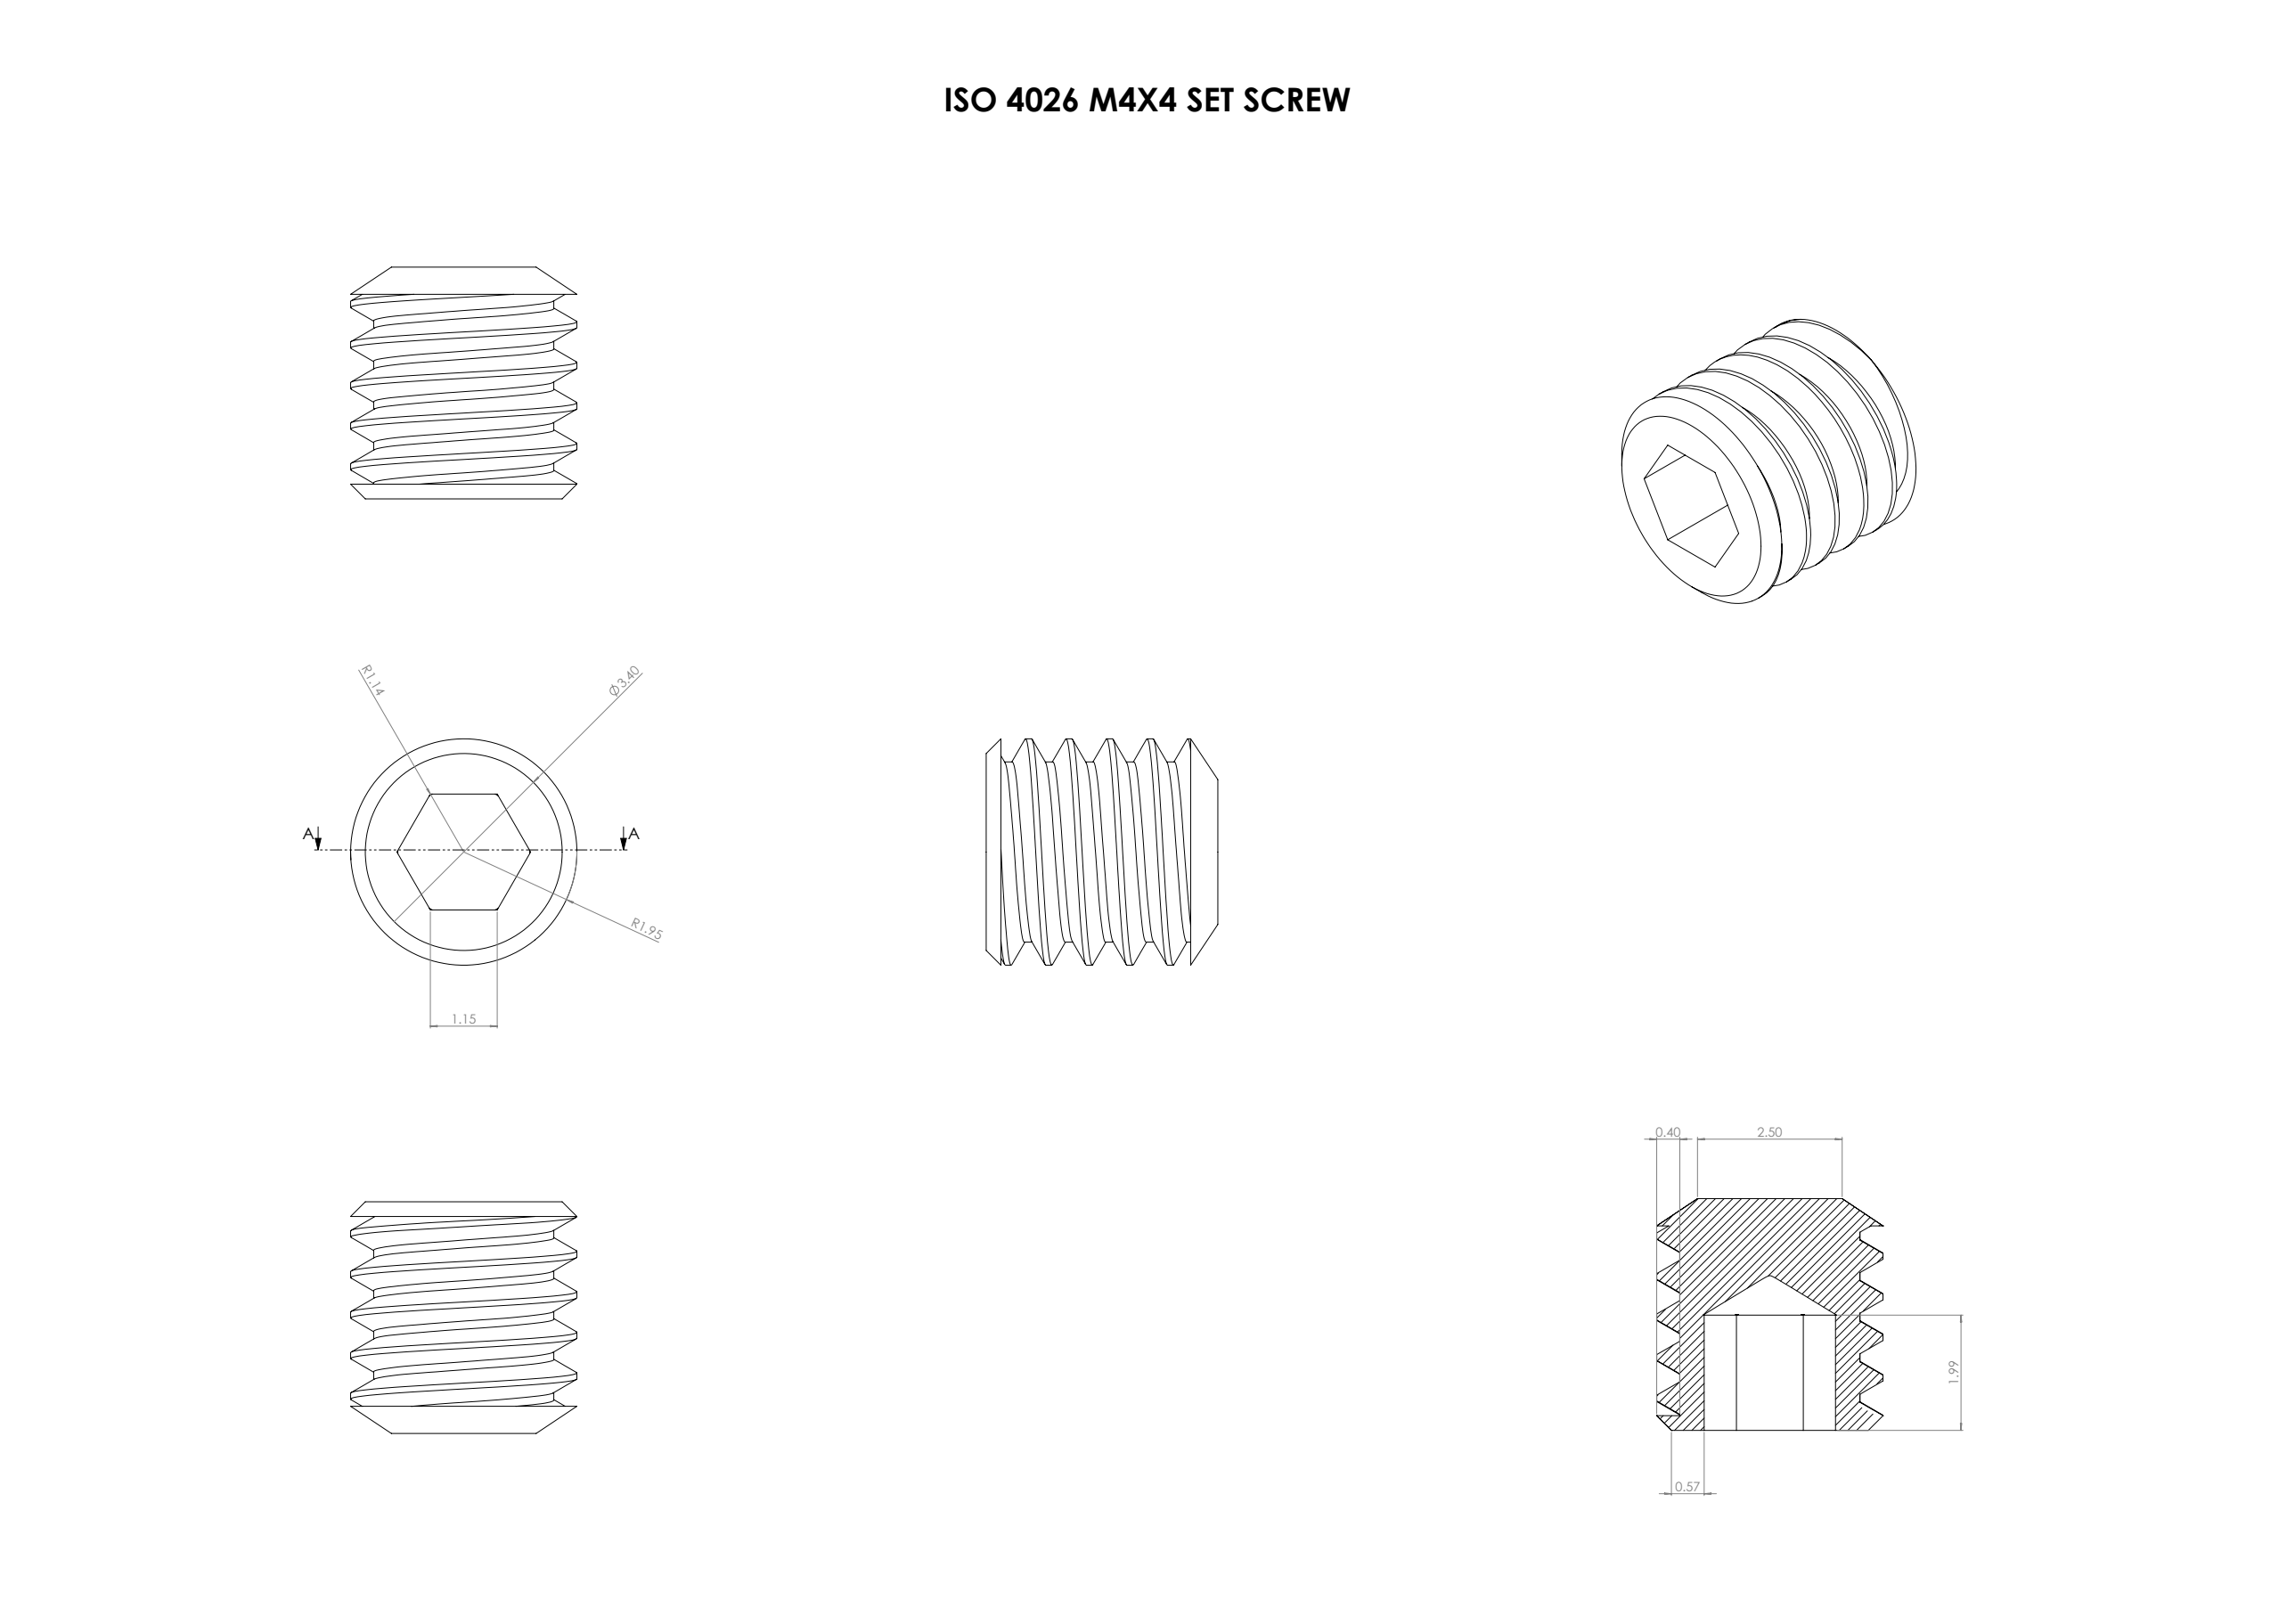
ISO-10303-21;
HEADER;
/* Generated by software containing ST-Developer
 * from STEP Tools, Inc. (www.steptools.com) 
 */

FILE_DESCRIPTION(
/* description */ (''),
/* implementation_level */ '2;1');

FILE_NAME(
/* name */ 
'14_ISO_4026_M4x4_Set_Screw.step',
/* time_stamp */ '2026-10-20T10:06:23-07:00',
/* author */ (''),
/* organization */ (''),
/* preprocessor_version */ 'ST-DEVELOPER v20.2',
/* originating_system */ 'Autodesk Translation Framework v15.15.0.0',
/* authorisation */ '');

FILE_SCHEMA (('AUTOMOTIVE_DESIGN { 1 0 10303 214 3 1 1 }'));
ENDSEC;

DATA;
#10=MECHANICAL_DESIGN_GEOMETRIC_PRESENTATION_REPRESENTATION('',(#467),#38611);
#118=(
BOUNDED_CURVE()
B_SPLINE_CURVE(2,(#26703,#26704,#26705),.UNSPECIFIED.,.F.,.F.)
B_SPLINE_CURVE_WITH_KNOTS((3,3),(0.,0.00350597452849922),.UNSPECIFIED.)
CURVE()
GEOMETRIC_REPRESENTATION_ITEM()
RATIONAL_B_SPLINE_CURVE((1.,1.00010739978215,1.))
REPRESENTATION_ITEM('')
);
#119=(
BOUNDED_CURVE()
B_SPLINE_CURVE(2,(#26707,#26708,#26709),.UNSPECIFIED.,.F.,.F.)
B_SPLINE_CURVE_WITH_KNOTS((3,3),(0.,0.00350597452849927),.UNSPECIFIED.)
CURVE()
GEOMETRIC_REPRESENTATION_ITEM()
RATIONAL_B_SPLINE_CURVE((1.,1.00010739978482,1.))
REPRESENTATION_ITEM('')
);
#120=(
BOUNDED_CURVE()
B_SPLINE_CURVE(2,(#26712,#26713,#26714),.UNSPECIFIED.,.F.,.F.)
B_SPLINE_CURVE_WITH_KNOTS((3,3),(0.,0.0035059745284993),.UNSPECIFIED.)
CURVE()
GEOMETRIC_REPRESENTATION_ITEM()
RATIONAL_B_SPLINE_CURVE((1.,1.00010739978303,1.))
REPRESENTATION_ITEM('')
);
#121=(
BOUNDED_CURVE()
B_SPLINE_CURVE(2,(#26716,#26717,#26718),.UNSPECIFIED.,.F.,.F.)
B_SPLINE_CURVE_WITH_KNOTS((3,3),(0.,0.00350597452849931),.UNSPECIFIED.)
CURVE()
GEOMETRIC_REPRESENTATION_ITEM()
RATIONAL_B_SPLINE_CURVE((1.,1.00010739978394,1.))
REPRESENTATION_ITEM('')
);
#122=(
BOUNDED_CURVE()
B_SPLINE_CURVE(2,(#26721,#26722,#26723),.UNSPECIFIED.,.F.,.F.)
B_SPLINE_CURVE_WITH_KNOTS((3,3),(0.,0.0035059745284993),.UNSPECIFIED.)
CURVE()
GEOMETRIC_REPRESENTATION_ITEM()
RATIONAL_B_SPLINE_CURVE((1.,1.00010739978631,1.))
REPRESENTATION_ITEM('')
);
#123=(
BOUNDED_CURVE()
B_SPLINE_CURVE(2,(#26725,#26726,#26727),.UNSPECIFIED.,.F.,.F.)
B_SPLINE_CURVE_WITH_KNOTS((3,3),(0.,0.00350597452849929),.UNSPECIFIED.)
CURVE()
GEOMETRIC_REPRESENTATION_ITEM()
RATIONAL_B_SPLINE_CURVE((1.,1.00010739978645,1.))
REPRESENTATION_ITEM('')
);
#124=(
BOUNDED_CURVE()
B_SPLINE_CURVE(2,(#26730,#26731,#26732),.UNSPECIFIED.,.F.,.F.)
B_SPLINE_CURVE_WITH_KNOTS((3,3),(0.,0.0035059745284993),.UNSPECIFIED.)
CURVE()
GEOMETRIC_REPRESENTATION_ITEM()
RATIONAL_B_SPLINE_CURVE((1.,1.00010739979569,1.))
REPRESENTATION_ITEM('')
);
#125=(
BOUNDED_CURVE()
B_SPLINE_CURVE(2,(#26734,#26735,#26736),.UNSPECIFIED.,.F.,.F.)
B_SPLINE_CURVE_WITH_KNOTS((3,3),(0.,0.0035059745284993),.UNSPECIFIED.)
CURVE()
GEOMETRIC_REPRESENTATION_ITEM()
RATIONAL_B_SPLINE_CURVE((1.,1.00010739979698,1.))
REPRESENTATION_ITEM('')
);
#126=(
BOUNDED_CURVE()
B_SPLINE_CURVE(2,(#26739,#26740,#26741),.UNSPECIFIED.,.F.,.F.)
B_SPLINE_CURVE_WITH_KNOTS((3,3),(0.,0.00350597452849928),.UNSPECIFIED.)
CURVE()
GEOMETRIC_REPRESENTATION_ITEM()
RATIONAL_B_SPLINE_CURVE((1.,1.00010739978256,1.))
REPRESENTATION_ITEM('')
);
#127=(
BOUNDED_CURVE()
B_SPLINE_CURVE(2,(#26743,#26744,#26745),.UNSPECIFIED.,.F.,.F.)
B_SPLINE_CURVE_WITH_KNOTS((3,3),(0.,0.00350597452849928),.UNSPECIFIED.)
CURVE()
GEOMETRIC_REPRESENTATION_ITEM()
RATIONAL_B_SPLINE_CURVE((1.,1.00010739978752,1.))
REPRESENTATION_ITEM('')
);
#128=(
BOUNDED_CURVE()
B_SPLINE_CURVE(2,(#26748,#26749,#26750),.UNSPECIFIED.,.F.,.F.)
B_SPLINE_CURVE_WITH_KNOTS((3,3),(0.,0.0035059745284993),.UNSPECIFIED.)
CURVE()
GEOMETRIC_REPRESENTATION_ITEM()
RATIONAL_B_SPLINE_CURVE((1.,1.0001073997843,1.))
REPRESENTATION_ITEM('')
);
#129=(
BOUNDED_CURVE()
B_SPLINE_CURVE(2,(#26752,#26753,#26754),.UNSPECIFIED.,.F.,.F.)
B_SPLINE_CURVE_WITH_KNOTS((3,3),(0.,0.00350597452849929),.UNSPECIFIED.)
CURVE()
GEOMETRIC_REPRESENTATION_ITEM()
RATIONAL_B_SPLINE_CURVE((1.,1.00010739978875,1.))
REPRESENTATION_ITEM('')
);
#439=SHAPE_REPRESENTATION_RELATIONSHIP('SRR','None',#38675,#453);
#453=ADVANCED_BREP_SHAPE_REPRESENTATION('',(#481),#38604);
#467=STYLED_ITEM('',(#38885),#481);
#481=MANIFOLD_SOLID_BREP('Set screw',#16241);
#499=B_SPLINE_SURFACE_WITH_KNOTS('',3,3,((#26238,#26239,#26240,#26241,#26242,
#26243,#26244,#26245,#26246,#26247,#26248,#26249,#26250,#26251,#26252,#26253,
#26254,#26255,#26256,#26257,#26258,#26259,#26260,#26261,#26262,#26263,#26264,
#26265,#26266,#26267,#26268,#26269,#26270,#26271,#26272),(#26273,#26274,
#26275,#26276,#26277,#26278,#26279,#26280,#26281,#26282,#26283,#26284,#26285,
#26286,#26287,#26288,#26289,#26290,#26291,#26292,#26293,#26294,#26295,#26296,
#26297,#26298,#26299,#26300,#26301,#26302,#26303,#26304,#26305,#26306,#26307),
(#26308,#26309,#26310,#26311,#26312,#26313,#26314,#26315,#26316,#26317,
#26318,#26319,#26320,#26321,#26322,#26323,#26324,#26325,#26326,#26327,#26328,
#26329,#26330,#26331,#26332,#26333,#26334,#26335,#26336,#26337,#26338,#26339,
#26340,#26341,#26342),(#26343,#26344,#26345,#26346,#26347,#26348,#26349,
#26350,#26351,#26352,#26353,#26354,#26355,#26356,#26357,#26358,#26359,#26360,
#26361,#26362,#26363,#26364,#26365,#26366,#26367,#26368,#26369,#26370,#26371,
#26372,#26373,#26374,#26375,#26376,#26377)),.UNSPECIFIED.,.F.,.F.,.F.,(4,
4),(4,1,1,1,1,1,1,1,1,1,1,1,1,1,1,1,1,1,1,1,1,1,1,1,1,1,1,1,1,1,1,1,4),
(0.,0.0460148164544132),(8.31058692273978,9.29422540264245,10.2778638825451,
11.2615023624478,12.2451408423505,13.2287793222531,14.2124178021558,15.1960562820585,
16.1796947619611,17.1633332418638,18.1469717217665,19.1306102016691,20.1142486815718,
21.0978871614745,22.0815256413772,23.0651641212798,24.0488026011825,25.0324410810852,
26.0160795609878,26.9997180408905,27.9833565207932,28.9669950006958,29.9506334805985,
30.9342719605012,31.9179104404039,32.9015489203065,33.8851874002092,34.8688258801119,
35.8524643600145,36.8361028399172,37.8197413198199,38.8033797997225,39.7870182796252),
 .UNSPECIFIED.);
#500=B_SPLINE_SURFACE_WITH_KNOTS('',3,3,((#26523,#26524,#26525,#26526,#26527,
#26528,#26529,#26530,#26531,#26532,#26533,#26534,#26535,#26536,#26537,#26538,
#26539,#26540,#26541,#26542,#26543,#26544,#26545,#26546,#26547,#26548,#26549,
#26550,#26551,#26552,#26553,#26554,#26555,#26556,#26557),(#26558,#26559,
#26560,#26561,#26562,#26563,#26564,#26565,#26566,#26567,#26568,#26569,#26570,
#26571,#26572,#26573,#26574,#26575,#26576,#26577,#26578,#26579,#26580,#26581,
#26582,#26583,#26584,#26585,#26586,#26587,#26588,#26589,#26590,#26591,#26592),
(#26593,#26594,#26595,#26596,#26597,#26598,#26599,#26600,#26601,#26602,
#26603,#26604,#26605,#26606,#26607,#26608,#26609,#26610,#26611,#26612,#26613,
#26614,#26615,#26616,#26617,#26618,#26619,#26620,#26621,#26622,#26623,#26624,
#26625,#26626,#26627),(#26628,#26629,#26630,#26631,#26632,#26633,#26634,
#26635,#26636,#26637,#26638,#26639,#26640,#26641,#26642,#26643,#26644,#26645,
#26646,#26647,#26648,#26649,#26650,#26651,#26652,#26653,#26654,#26655,#26656,
#26657,#26658,#26659,#26660,#26661,#26662)),.UNSPECIFIED.,.F.,.F.,.F.,(4,
4),(4,1,1,1,1,1,1,1,1,1,1,1,1,1,1,1,1,1,1,1,1,1,1,1,1,1,1,1,1,1,1,1,4),
(0.,0.0460148164544132),(11.6154215191106,12.5990599990133,13.582698478916,
14.5663369588187,15.5499754387213,16.533613918624,17.5172523985267,18.5008908784293,
19.484529358332,20.4681678382347,21.4518063181373,22.43544479804,23.4190832779427,
24.4027217578453,25.386360237748,26.3699987176507,27.3536371975534,28.337275677456,
29.3209141573587,30.3045526372614,31.288191117164,32.2718295970667,33.2554680769694,
34.239106556872,35.2227450367747,36.2063835166774,37.19002199658,38.1736604764827,
39.1572989563854,40.1409374362881,41.1245759161907,42.1082143960934,43.0918528759961),
 .UNSPECIFIED.);
#592=B_SPLINE_CURVE_WITH_KNOTS('',3,(#25799,#25800,#25801,#25802,#25803,
#25804,#25805,#25806,#25807,#25808),.UNSPECIFIED.,.F.,.F.,(4,3,3,4),(-4.09254174883832,
-3.93455391961068,-2.95091543970801,-2.06514013327811),.UNSPECIFIED.);
#593=B_SPLINE_CURVE_WITH_KNOTS('',3,(#25811,#25812,#25813,#25814,#25815,
#25816,#25817),.UNSPECIFIED.,.F.,.F.,(4,3,4),(0.,0.983638479902673,1.11419103802959),
 .UNSPECIFIED.);
#594=B_SPLINE_CURVE_WITH_KNOTS('',3,(#25822,#25823,#25824,#25825,#25826,
#25827,#25828,#25829,#25830,#25831,#25832,#25833,#25834,#25835,#25836,#25837,
#25838,#25839,#25840,#25841,#25842,#25843),.UNSPECIFIED.,.F.,.F.,(4,3,3,
3,3,3,3,4),(-10.3757270560179,-9.83638479902669,-8.85274631912402,-7.86910783922136,
-6.88546935931869,-5.90183087941602,-4.91819239951335,-4.09254174883832),
 .UNSPECIFIED.);
#595=B_SPLINE_CURVE_WITH_KNOTS('',3,(#25844,#25845,#25846,#25847,#25848,
#25849,#25850,#25851,#25852,#25853,#25854,#25855,#25856,#25857,#25858,#25859,
#25860,#25861,#25862,#25863,#25864,#25865),.UNSPECIFIED.,.F.,.F.,(4,3,3,
3,3,3,3,4),(1.11419103802959,1.96727695980534,2.95091543970801,3.93455391961068,
4.91819239951335,5.90183087941602,6.88546935931869,7.39737634520918),
 .UNSPECIFIED.);
#596=B_SPLINE_CURVE_WITH_KNOTS('',3,(#25870,#25871,#25872,#25873,#25874,
#25875,#25876,#25877,#25878,#25879,#25880,#25881,#25882,#25883,#25884,#25885,
#25886,#25887,#25888,#25889,#25890,#25891),.UNSPECIFIED.,.F.,.F.,(4,3,3,
3,3,3,3,4),(-16.6589123631975,-15.7382156784427,-14.75457719854,-13.7709387186374,
-12.7873002387347,-11.803661758832,-10.8200232789294,-10.3757270560179),
 .UNSPECIFIED.);
#597=B_SPLINE_CURVE_WITH_KNOTS('',3,(#25892,#25893,#25894,#25895,#25896,
#25897,#25898,#25899,#25900,#25901,#25902,#25903,#25904,#25905,#25906,#25907,
#25908,#25909,#25910,#25911,#25912,#25913),.UNSPECIFIED.,.F.,.F.,(4,3,3,
3,3,3,3,4),(7.39737634520918,7.86910783922136,8.85274631912403,9.83638479902669,
10.8200232789294,11.803661758832,12.7873002387347,13.6805616523888),
 .UNSPECIFIED.);
#598=B_SPLINE_CURVE_WITH_KNOTS('',3,(#25918,#25919,#25920,#25921,#25922,
#25923,#25924,#25925,#25926,#25927,#25928,#25929,#25930,#25931,#25932,#25933,
#25934,#25935,#25936,#25937,#25938,#25939,#25940,#25941,#25942),
 .UNSPECIFIED.,.F.,.F.,(4,3,3,3,3,3,3,3,4),(-22.9420976703771,-22.6236850377614,
-21.6400465578587,-20.6564080779561,-19.6727695980534,-18.6891311181507,
-17.705492638248,-16.7218541583454,-16.6589123631975),.UNSPECIFIED.);
#599=B_SPLINE_CURVE_WITH_KNOTS('',3,(#25943,#25944,#25945,#25946,#25947,
#25948,#25949,#25950,#25951,#25952,#25953,#25954,#25955,#25956,#25957,#25958,
#25959,#25960,#25961,#25962,#25963,#25964,#25965,#25966,#25967),
 .UNSPECIFIED.,.F.,.F.,(4,3,3,3,3,3,3,3,4),(13.6805616523888,13.7709387186374,
14.75457719854,15.7382156784427,16.7218541583454,17.705492638248,18.6891311181507,
19.6727695980534,19.9637469595684),.UNSPECIFIED.);
#600=B_SPLINE_CURVE_WITH_KNOTS('',3,(#25972,#25973,#25974,#25975,#25976,
#25977,#25978,#25979,#25980,#25981,#25982,#25983,#25984,#25985,#25986,#25987,
#25988,#25989,#25990,#25991,#25992,#25993),.UNSPECIFIED.,.F.,.F.,(4,3,3,
3,3,3,3,4),(-29.2252829775567,-28.5255159171774,-27.5418774372747,-26.5582389573721,
-25.5746004774694,-24.5909619975667,-23.6073235176641,-22.9420976703771),
 .UNSPECIFIED.);
#601=B_SPLINE_CURVE_WITH_KNOTS('',3,(#25994,#25995,#25996,#25997,#25998,
#25999,#26000,#26001,#26002,#26003,#26004,#26005,#26006,#26007,#26008,#26009,
#26010,#26011,#26012,#26013,#26014,#26015),.UNSPECIFIED.,.F.,.F.,(4,3,3,
3,3,3,3,4),(19.9637469595684,20.6564080779561,21.6400465578587,22.6236850377614,
23.6073235176641,24.5909619975667,25.5746004774694,26.2469322667479),
 .UNSPECIFIED.);
#602=B_SPLINE_CURVE_WITH_KNOTS('',3,(#26021,#26022,#26023,#26024),
 .UNSPECIFIED.,.F.,.F.,(4,4),(40.8407044966673,41.026712742718),
 .UNSPECIFIED.);
#603=B_SPLINE_CURVE_WITH_KNOTS('',3,(#26030,#26031,#26032,#26033,#26034,
#26035,#26036,#26037,#26038,#26039),.UNSPECIFIED.,.F.,.F.,(4,1,1,1,1,1,
1,4),(34.5575191894877,35.2227450367747,36.2063835166774,37.19002199658,
38.1736604764827,39.1572989563854,40.1409374362881,40.8407044966673),
 .UNSPECIFIED.);
#604=B_SPLINE_CURVE_WITH_KNOTS('',3,(#26042,#26043,#26044,#26045,#26046,
#26047,#26048,#26049,#26050),.UNSPECIFIED.,.F.,.F.,(4,1,1,1,1,1,4),(34.5575191894877,
34.8688258801119,35.8524643600145,36.8361028399172,37.8197413198199,38.8033797997225,
39.7870182796252),.UNSPECIFIED.);
#605=B_SPLINE_CURVE_WITH_KNOTS('',3,(#26055,#26056,#26057,#26058,#26059,
#26060,#26061,#26062,#26063,#26064,#26065),.UNSPECIFIED.,.F.,.F.,(4,1,1,
1,1,1,1,1,4),(28.2743338823081,28.337275677456,29.3209141573587,30.3045526372614,
31.288191117164,32.2718295970667,33.2554680769694,34.239106556872,34.5575191894877),
 .UNSPECIFIED.);
#606=B_SPLINE_CURVE_WITH_KNOTS('',3,(#26066,#26067,#26068,#26069,#26070,
#26071,#26072,#26073,#26074,#26075),.UNSPECIFIED.,.F.,.F.,(4,1,1,1,1,1,
1,4),(28.2743338823081,28.9669950006958,29.9506334805985,30.9342719605012,
31.9179104404039,32.9015489203065,33.8851874002092,34.5575191894877),
 .UNSPECIFIED.);
#607=B_SPLINE_CURVE_WITH_KNOTS('',3,(#26080,#26081,#26082,#26083,#26084,
#26085,#26086,#26087,#26088,#26089),.UNSPECIFIED.,.F.,.F.,(4,1,1,1,1,1,
1,4),(21.9911485751285,22.43544479804,23.4190832779427,24.4027217578453,
25.386360237748,26.3699987176507,27.3536371975534,28.2743338823081),
 .UNSPECIFIED.);
#608=B_SPLINE_CURVE_WITH_KNOTS('',3,(#26090,#26091,#26092,#26093,#26094,
#26095,#26096,#26097,#26098,#26099,#26100),.UNSPECIFIED.,.F.,.F.,(4,1,1,
1,1,1,1,1,4),(21.9911485751285,22.0815256413772,23.0651641212798,24.0488026011825,
25.0324410810852,26.0160795609878,26.9997180408905,27.9833565207932,28.2743338823081),
 .UNSPECIFIED.);
#609=B_SPLINE_CURVE_WITH_KNOTS('',3,(#26105,#26106,#26107,#26108,#26109,
#26110,#26111,#26112,#26113,#26114),.UNSPECIFIED.,.F.,.F.,(4,1,1,1,1,1,
1,4),(15.707963267949,16.533613918624,17.5172523985267,18.5008908784293,
19.484529358332,20.4681678382347,21.4518063181373,21.9911485751285),
 .UNSPECIFIED.);
#610=B_SPLINE_CURVE_WITH_KNOTS('',3,(#26115,#26116,#26117,#26118,#26119,
#26120,#26121,#26122,#26123,#26124),.UNSPECIFIED.,.F.,.F.,(4,1,1,1,1,1,
1,4),(15.707963267949,16.1796947619611,17.1633332418638,18.1469717217665,
19.1306102016691,20.1142486815718,21.0978871614745,21.9911485751285),
 .UNSPECIFIED.);
#611=B_SPLINE_CURVE_WITH_KNOTS('',3,(#26127,#26128,#26129,#26130,#26131,
#26132,#26133,#26134,#26135,#26136,#26137,#26138,#26139,#26140,#26141,#26142,
#26143,#26144,#26145,#26146,#26147,#26148,#26149,#26150,#26151,#26152,#26153,
#26154,#26155,#26156,#26157,#26158,#26159,#26160,#26161,#26162,#26163,#26164,
#26165,#26166,#26167,#26168,#26169,#26170,#26171,#26172,#26173,#26174,#26175,
#26176,#26177,#26178),.UNSPECIFIED.,.F.,.F.,(4,3,3,3,3,3,3,3,3,3,3,3,3,
3,3,3,3,4),(-0.366397579005848,-0.350883706971702,-0.330766239349036,-0.315517000142461,
-0.286726965402577,-0.272902702918689,-0.237792065049709,-0.221751325260965,
-0.207725190445974,-0.184643803987141,-0.160983363133761,-0.147813025816132,
-0.137069449159236,-0.102802086869427,-0.0797357051045986,-0.0678496931522027,
-0.0293463862030034,0.),.UNSPECIFIED.);
#612=B_SPLINE_CURVE_WITH_KNOTS('',3,(#26183,#26184,#26185,#26186,#26187,
#26188,#26189,#26190,#26191,#26192,#26193,#26194,#26195,#26196,#26197,#26198,
#26199,#26200,#26201,#26202,#26203,#26204,#26205,#26206,#26207,#26208,#26209,
#26210,#26211,#26212,#26213,#26214,#26215,#26216,#26217,#26218,#26219,#26220,
#26221,#26222,#26223,#26224,#26225,#26226,#26227,#26228,#26229,#26230,#26231,
#26232,#26233,#26234,#26235,#26236,#26237),.UNSPECIFIED.,.F.,.F.,(4,3,3,
3,3,3,3,3,3,3,3,3,3,3,3,3,3,3,4),(-0.364629307890673,-0.34556327172486,
-0.316373806239452,-0.304392727635835,-0.282581484008551,-0.264372375760159,
-0.252241992724549,-0.215817384559742,-0.198585804821849,-0.187223821335194,
-0.163761333129925,-0.14297227179632,-0.127520914102002,-0.116250236265464,
-0.0871876771990984,-0.0683674864494023,-0.0546742414735358,-0.0223329481946053,
0.),.UNSPECIFIED.);
#613=B_SPLINE_CURVE_WITH_KNOTS('',3,(#26378,#26379,#26380,#26381,#26382,
#26383,#26384,#26385,#26386,#26387,#26388,#26389,#26390),.UNSPECIFIED.,
 .F.,.F.,(4,3,3,3,4),(26.2469322667479,26.5582389573721,27.5418774372747,
28.5255159171774,29.4112912236073),.UNSPECIFIED.);
#614=B_SPLINE_CURVE_WITH_KNOTS('',3,(#26392,#26393,#26394,#26395,#26396,
#26397,#26398,#26399,#26400,#26401,#26402,#26403,#26404,#26405,#26406,#26407,
#26408,#26409,#26410,#26411,#26412,#26413,#26414,#26415,#26416,#26417,#26418,
#26419,#26420,#26421,#26422,#26423,#26424,#26425,#26426,#26427,#26428,#26429,
#26430,#26431,#26432,#26433,#26434,#26435,#26436,#26437,#26438,#26439,#26440,
#26441,#26442,#26443),.UNSPECIFIED.,.F.,.F.,(4,3,3,3,3,3,3,3,3,3,3,3,3,
3,3,3,3,4),(-0.366397579005841,-0.350883706971692,-0.330766244233555,-0.315517008906463,
-0.286727928129561,-0.272902925597775,-0.237792297289449,-0.221751641342226,
-0.207725209589122,-0.184643803987137,-0.160983359465905,-0.147812972159593,
-0.137069363910321,-0.102802022932741,-0.0797355322205692,-0.0678497129848781,
-0.0293463878428536,0.),.UNSPECIFIED.);
#615=B_SPLINE_CURVE_WITH_KNOTS('',3,(#26444,#26445,#26446,#26447,#26448,
#26449,#26450,#26451,#26452),.UNSPECIFIED.,.F.,.F.,(4,1,1,1,1,1,4),(10.3757270560179,
11.2615023624478,12.2451408423505,13.2287793222531,14.2124178021558,15.1960562820585,
15.707963267949),.UNSPECIFIED.);
#616=B_SPLINE_CURVE_WITH_KNOTS('',3,(#26458,#26459,#26460,#26461,#26462,
#26463,#26464,#26465,#26466,#26467,#26468,#26469,#26470,#26471,#26472,#26473,
#26474,#26475,#26476,#26477,#26478,#26479,#26480,#26481,#26482,#26483,#26484,
#26485,#26486,#26487,#26488,#26489,#26490,#26491,#26492,#26493,#26494,#26495,
#26496,#26497,#26498,#26499,#26500,#26501,#26502,#26503,#26504,#26505,#26506,
#26507,#26508,#26509,#26510,#26511,#26512),.UNSPECIFIED.,.F.,.F.,(4,3,3,
3,3,3,3,3,3,3,3,3,3,3,3,3,3,3,4),(-0.364629307890667,-0.345563271724857,
-0.316373785930453,-0.304392687069709,-0.282581361533379,-0.264370838693491,
-0.252241562212899,-0.215816938962755,-0.198585271532288,-0.18722386611403,
-0.163761333129928,-0.142972181196261,-0.127520768604021,-0.116250225520689,
-0.087187669140517,-0.0683674708033287,-0.0546742449026845,-0.0223330177554359,
0.),.UNSPECIFIED.);
#617=B_SPLINE_CURVE_WITH_KNOTS('',3,(#26515,#26516,#26517,#26518,#26519,
#26520,#26521,#26522),.UNSPECIFIED.,.F.,.F.,(4,1,1,1,1,4),(11.6154215191106,
12.5990599990133,13.582698478916,14.5663369588187,15.5499754387213,15.707963267949),
 .UNSPECIFIED.);
#618=B_SPLINE_CURVE_WITH_KNOTS('',3,(#26663,#26664,#26665,#26666,#26667,
#26668,#26669,#26670,#26671,#26672),.UNSPECIFIED.,.F.,.F.,(4,3,3,4),(-31.4764313568854,
-30.4927928769827,-29.5091543970801,-29.2252829775567),.UNSPECIFIED.);
#930=CYLINDRICAL_SURFACE('',#16910,0.1954);
#931=CYLINDRICAL_SURFACE('',#16912,0.1954);
#932=CYLINDRICAL_SURFACE('',#16913,0.1954);
#933=CYLINDRICAL_SURFACE('',#16914,0.1954);
#934=CYLINDRICAL_SURFACE('',#16915,0.1954);
#935=CYLINDRICAL_SURFACE('',#16916,0.15555);
#936=CYLINDRICAL_SURFACE('',#16918,0.15555);
#937=CYLINDRICAL_SURFACE('',#16920,0.15555);
#938=CYLINDRICAL_SURFACE('',#16921,0.15555);
#939=CYLINDRICAL_SURFACE('',#16922,0.15555);
#940=CYLINDRICAL_SURFACE('',#16930,0.15555);
#941=CYLINDRICAL_SURFACE('',#16978,0.1954);
#1187=FACE_BOUND('',#3096,.T.);
#1386=CIRCLE('',#16911,0.1954);
#1387=CIRCLE('',#16917,0.15555);
#1388=CIRCLE('',#16919,0.15555);
#1389=CIRCLE('',#16924,0.1954);
#1390=CIRCLE('',#16925,0.1954);
#1391=CIRCLE('',#16927,0.1954);
#1392=CIRCLE('',#16928,0.1954);
#1393=CIRCLE('',#16929,0.15555);
#1394=CIRCLE('',#16932,0.115470053837925);
#1395=CIRCLE('',#16934,0.115470053837925);
#1396=CIRCLE('',#16936,0.115470053837925);
#1397=CIRCLE('',#16938,0.115470053837925);
#1398=CIRCLE('',#16940,0.115470053837925);
#1399=CIRCLE('',#16942,0.115470053837925);
#1400=CIRCLE('',#16944,0.113827101150665);
#1401=CIRCLE('',#16945,0.113827101150665);
#1402=CIRCLE('',#16946,0.113827101150665);
#1403=CIRCLE('',#16947,0.113827101150665);
#1404=CIRCLE('',#16948,0.113827101150665);
#1405=CIRCLE('',#16949,0.113827101150665);
#1406=CIRCLE('',#16950,0.113827101150665);
#1407=CIRCLE('',#16976,0.125);
#1408=CIRCLE('',#16979,0.1954);
#1409=CIRCLE('',#16981,0.17);
#1743=CONICAL_SURFACE('',#16943,0.0577350269189626,1.02403331474479);
#1744=CONICAL_SURFACE('',#16977,0.1625,0.982793723247329);
#1745=CONICAL_SURFACE('',#16980,0.185,0.785398163397449);
#2100=FACE_OUTER_BOUND('',#3045,.T.);
#2101=FACE_OUTER_BOUND('',#3046,.T.);
#2102=FACE_OUTER_BOUND('',#3047,.T.);
#2103=FACE_OUTER_BOUND('',#3048,.T.);
#2104=FACE_OUTER_BOUND('',#3049,.T.);
#2105=FACE_OUTER_BOUND('',#3050,.T.);
#2106=FACE_OUTER_BOUND('',#3051,.T.);
#2107=FACE_OUTER_BOUND('',#3052,.T.);
#2108=FACE_OUTER_BOUND('',#3053,.T.);
#2109=FACE_OUTER_BOUND('',#3054,.T.);
#2110=FACE_OUTER_BOUND('',#3055,.T.);
#2111=FACE_OUTER_BOUND('',#3056,.T.);
#2112=FACE_OUTER_BOUND('',#3057,.T.);
#2113=FACE_OUTER_BOUND('',#3058,.T.);
#2114=FACE_OUTER_BOUND('',#3059,.T.);
#2115=FACE_OUTER_BOUND('',#3060,.T.);
#2116=FACE_OUTER_BOUND('',#3061,.T.);
#2117=FACE_OUTER_BOUND('',#3062,.T.);
#2118=FACE_OUTER_BOUND('',#3063,.T.);
#2119=FACE_OUTER_BOUND('',#3064,.T.);
#2120=FACE_OUTER_BOUND('',#3065,.T.);
#2121=FACE_OUTER_BOUND('',#3066,.T.);
#2122=FACE_OUTER_BOUND('',#3067,.T.);
#2123=FACE_OUTER_BOUND('',#3068,.T.);
#2124=FACE_OUTER_BOUND('',#3069,.T.);
#2125=FACE_OUTER_BOUND('',#3070,.T.);
#2126=FACE_OUTER_BOUND('',#3071,.T.);
#2127=FACE_OUTER_BOUND('',#3072,.T.);
#2128=FACE_OUTER_BOUND('',#3073,.T.);
#2129=FACE_OUTER_BOUND('',#3074,.T.);
#2130=FACE_OUTER_BOUND('',#3075,.T.);
#2131=FACE_OUTER_BOUND('',#3076,.T.);
#2132=FACE_OUTER_BOUND('',#3077,.T.);
#2133=FACE_OUTER_BOUND('',#3078,.T.);
#2134=FACE_OUTER_BOUND('',#3079,.T.);
#2135=FACE_OUTER_BOUND('',#3080,.T.);
#2136=FACE_OUTER_BOUND('',#3081,.T.);
#2137=FACE_OUTER_BOUND('',#3082,.T.);
#2138=FACE_OUTER_BOUND('',#3083,.T.);
#2139=FACE_OUTER_BOUND('',#3084,.T.);
#2140=FACE_OUTER_BOUND('',#3085,.T.);
#2141=FACE_OUTER_BOUND('',#3086,.T.);
#2142=FACE_OUTER_BOUND('',#3087,.T.);
#2143=FACE_OUTER_BOUND('',#3088,.T.);
#2144=FACE_OUTER_BOUND('',#3089,.T.);
#2145=FACE_OUTER_BOUND('',#3090,.T.);
#2146=FACE_OUTER_BOUND('',#3091,.T.);
#2147=FACE_OUTER_BOUND('',#3092,.T.);
#2148=FACE_OUTER_BOUND('',#3093,.T.);
#2149=FACE_OUTER_BOUND('',#3094,.T.);
#2150=FACE_OUTER_BOUND('',#3095,.T.);
#3045=EDGE_LOOP('',(#11601,#11602,#11603,#11604));
#3046=EDGE_LOOP('',(#11605,#11606,#11607,#11608));
#3047=EDGE_LOOP('',(#11609,#11610,#11611,#11612));
#3048=EDGE_LOOP('',(#11613,#11614,#11615,#11616));
#3049=EDGE_LOOP('',(#11617,#11618,#11619,#11620));
#3050=EDGE_LOOP('',(#11621,#11622,#11623));
#3051=EDGE_LOOP('',(#11624,#11625,#11626,#11627,#11628));
#3052=EDGE_LOOP('',(#11629,#11630,#11631,#11632));
#3053=EDGE_LOOP('',(#11633,#11634,#11635,#11636));
#3054=EDGE_LOOP('',(#11637,#11638,#11639,#11640));
#3055=EDGE_LOOP('',(#11641,#11642,#11643,#11644,#11645,#11646));
#3056=EDGE_LOOP('',(#11647,#11648,#11649,#11650,#11651,#11652,#11653,#11654,
#11655,#11656,#11657,#11658,#11659));
#3057=EDGE_LOOP('',(#11660,#11661,#11662,#11663,#11664));
#3058=EDGE_LOOP('',(#11665,#11666,#11667,#11668));
#3059=EDGE_LOOP('',(#11669,#11670,#11671,#11672,#11673,#11674,#11675,#11676,
#11677,#11678,#11679,#11680,#11681,#11682));
#3060=EDGE_LOOP('',(#11683,#11684));
#3061=EDGE_LOOP('',(#11685,#11686));
#3062=EDGE_LOOP('',(#11687,#11688));
#3063=EDGE_LOOP('',(#11689,#11690));
#3064=EDGE_LOOP('',(#11691,#11692));
#3065=EDGE_LOOP('',(#11693,#11694));
#3066=EDGE_LOOP('',(#11695,#11696,#11697,#11698,#11699,#11700,#11701,#11702,
#11703,#11704,#11705,#11706,#11707,#11708,#11709,#11710,#11711,#11712,#11713,
#11714,#11715,#11716,#11717,#11718,#11719,#11720,#11721));
#3067=EDGE_LOOP('',(#11722,#11723,#11724,#11725));
#3068=EDGE_LOOP('',(#11726,#11727,#11728));
#3069=EDGE_LOOP('',(#11729,#11730,#11731,#11732));
#3070=EDGE_LOOP('',(#11733,#11734,#11735));
#3071=EDGE_LOOP('',(#11736,#11737,#11738));
#3072=EDGE_LOOP('',(#11739,#11740,#11741,#11742));
#3073=EDGE_LOOP('',(#11743,#11744,#11745));
#3074=EDGE_LOOP('',(#11746,#11747,#11748,#11749));
#3075=EDGE_LOOP('',(#11750,#11751,#11752));
#3076=EDGE_LOOP('',(#11753,#11754,#11755));
#3077=EDGE_LOOP('',(#11756,#11757,#11758));
#3078=EDGE_LOOP('',(#11759,#11760,#11761));
#3079=EDGE_LOOP('',(#11762,#11763,#11764));
#3080=EDGE_LOOP('',(#11765,#11766,#11767));
#3081=EDGE_LOOP('',(#11768,#11769,#11770));
#3082=EDGE_LOOP('',(#11771,#11772,#11773,#11774));
#3083=EDGE_LOOP('',(#11775,#11776,#11777,#11778));
#3084=EDGE_LOOP('',(#11779,#11780,#11781));
#3085=EDGE_LOOP('',(#11782,#11783,#11784));
#3086=EDGE_LOOP('',(#11785,#11786,#11787));
#3087=EDGE_LOOP('',(#11788,#11789,#11790,#11791));
#3088=EDGE_LOOP('',(#11792,#11793,#11794));
#3089=EDGE_LOOP('',(#11795,#11796,#11797));
#3090=EDGE_LOOP('',(#11798,#11799,#11800));
#3091=EDGE_LOOP('',(#11801));
#3092=EDGE_LOOP('',(#11802,#11803,#11804,#11805,#11806,#11807));
#3093=EDGE_LOOP('',(#11808,#11809,#11810,#11811));
#3094=EDGE_LOOP('',(#11812,#11813,#11814,#11815,#11816,#11817));
#3095=EDGE_LOOP('',(#11818));
#3096=EDGE_LOOP('',(#11819,#11820,#11821,#11822,#11823,#11824));
#4162=LINE('',#25797,#5386);
#4163=LINE('',#25821,#5387);
#4164=LINE('',#25869,#5388);
#4165=LINE('',#25917,#5389);
#4166=LINE('',#25971,#5390);
#4167=LINE('',#26019,#5391);
#4168=LINE('',#26029,#5392);
#4169=LINE('',#26054,#5393);
#4170=LINE('',#26079,#5394);
#4171=LINE('',#26104,#5395);
#4172=LINE('',#26676,#5396);
#4173=LINE('',#26680,#5397);
#4174=LINE('',#26684,#5398);
#4175=LINE('',#26688,#5399);
#4176=LINE('',#26692,#5400);
#4177=LINE('',#26695,#5401);
#4178=LINE('',#26700,#5402);
#4179=LINE('',#26758,#5403);
#4180=LINE('',#26760,#5404);
#4181=LINE('',#26761,#5405);
#4182=LINE('',#26764,#5406);
#4183=LINE('',#26765,#5407);
#4184=LINE('',#26768,#5408);
#4185=LINE('',#26769,#5409);
#4186=LINE('',#26772,#5410);
#4187=LINE('',#26773,#5411);
#4188=LINE('',#26776,#5412);
#4189=LINE('',#26777,#5413);
#4190=LINE('',#26780,#5414);
#4191=LINE('',#26781,#5415);
#4192=LINE('',#26784,#5416);
#4193=LINE('',#26785,#5417);
#4194=LINE('',#26788,#5418);
#4195=LINE('',#26789,#5419);
#4196=LINE('',#26792,#5420);
#4197=LINE('',#26793,#5421);
#4198=LINE('',#26795,#5422);
#4199=LINE('',#26797,#5423);
#4200=LINE('',#26800,#5424);
#4201=LINE('',#26803,#5425);
#4202=LINE('',#26804,#5426);
#4203=LINE('',#26806,#5427);
#4204=LINE('',#26808,#5428);
#4205=LINE('',#26811,#5429);
#4206=LINE('',#26812,#5430);
#4207=LINE('',#26814,#5431);
#4208=LINE('',#26818,#5432);
#4209=LINE('',#26826,#5433);
#4210=LINE('',#26832,#5434);
#5386=VECTOR('',#19329,0.2);
#5387=VECTOR('',#19334,0.2);
#5388=VECTOR('',#19337,0.2);
#5389=VECTOR('',#19340,0.2);
#5390=VECTOR('',#19343,0.2);
#5391=VECTOR('',#19346,0.15555);
#5392=VECTOR('',#19351,0.15555);
#5393=VECTOR('',#19356,0.15555);
#5394=VECTOR('',#19359,0.15555);
#5395=VECTOR('',#19362,0.15555);
#5396=VECTOR('',#19381,1.);
#5397=VECTOR('',#19386,1.);
#5398=VECTOR('',#19391,1.);
#5399=VECTOR('',#19396,1.);
#5400=VECTOR('',#19401,1.);
#5401=VECTOR('',#19406,1.);
#5402=VECTOR('',#19411,0.0577350269189626);
#5403=VECTOR('',#19428,1.);
#5404=VECTOR('',#19429,1.);
#5405=VECTOR('',#19430,1.);
#5406=VECTOR('',#19433,1.);
#5407=VECTOR('',#19434,1.);
#5408=VECTOR('',#19437,1.);
#5409=VECTOR('',#19438,1.);
#5410=VECTOR('',#19441,1.);
#5411=VECTOR('',#19442,1.);
#5412=VECTOR('',#19445,1.);
#5413=VECTOR('',#19446,1.);
#5414=VECTOR('',#19449,1.);
#5415=VECTOR('',#19450,1.);
#5416=VECTOR('',#19453,1.);
#5417=VECTOR('',#19454,1.);
#5418=VECTOR('',#19457,1.);
#5419=VECTOR('',#19458,1.);
#5420=VECTOR('',#19461,1.);
#5421=VECTOR('',#19462,1.);
#5422=VECTOR('',#19465,1.);
#5423=VECTOR('',#19468,1.);
#5424=VECTOR('',#19473,1.);
#5425=VECTOR('',#19476,1.);
#5426=VECTOR('',#19477,1.);
#5427=VECTOR('',#19480,1.);
#5428=VECTOR('',#19483,1.);
#5429=VECTOR('',#19486,1.);
#5430=VECTOR('',#19487,1.);
#5431=VECTOR('',#19490,1.);
#5432=VECTOR('',#19497,1.);
#5433=VECTOR('',#19510,0.1625);
#5434=VECTOR('',#19519,0.185);
#6589=VERTEX_POINT('',#25795);
#6590=VERTEX_POINT('',#25796);
#6591=VERTEX_POINT('',#25798);
#6592=VERTEX_POINT('',#25809);
#6593=VERTEX_POINT('',#25819);
#6594=VERTEX_POINT('',#25820);
#6595=VERTEX_POINT('',#25867);
#6596=VERTEX_POINT('',#25868);
#6597=VERTEX_POINT('',#25915);
#6598=VERTEX_POINT('',#25916);
#6599=VERTEX_POINT('',#25969);
#6600=VERTEX_POINT('',#25970);
#6601=VERTEX_POINT('',#26017);
#6602=VERTEX_POINT('',#26018);
#6603=VERTEX_POINT('',#26020);
#6604=VERTEX_POINT('',#26027);
#6605=VERTEX_POINT('',#26028);
#6606=VERTEX_POINT('',#26040);
#6607=VERTEX_POINT('',#26052);
#6608=VERTEX_POINT('',#26053);
#6609=VERTEX_POINT('',#26077);
#6610=VERTEX_POINT('',#26078);
#6611=VERTEX_POINT('',#26102);
#6612=VERTEX_POINT('',#26103);
#6613=VERTEX_POINT('',#26126);
#6614=VERTEX_POINT('',#26179);
#6615=VERTEX_POINT('',#26181);
#6616=VERTEX_POINT('',#26391);
#6617=VERTEX_POINT('',#26454);
#6618=VERTEX_POINT('',#26457);
#6619=VERTEX_POINT('',#26674);
#6620=VERTEX_POINT('',#26675);
#6621=VERTEX_POINT('',#26679);
#6622=VERTEX_POINT('',#26683);
#6623=VERTEX_POINT('',#26687);
#6624=VERTEX_POINT('',#26691);
#6625=VERTEX_POINT('',#26698);
#6626=VERTEX_POINT('',#26699);
#6627=VERTEX_POINT('',#26701);
#6628=VERTEX_POINT('',#26706);
#6629=VERTEX_POINT('',#26710);
#6630=VERTEX_POINT('',#26715);
#6631=VERTEX_POINT('',#26719);
#6632=VERTEX_POINT('',#26724);
#6633=VERTEX_POINT('',#26728);
#6634=VERTEX_POINT('',#26733);
#6635=VERTEX_POINT('',#26737);
#6636=VERTEX_POINT('',#26742);
#6637=VERTEX_POINT('',#26746);
#6638=VERTEX_POINT('',#26751);
#6639=VERTEX_POINT('',#26757);
#6640=VERTEX_POINT('',#26759);
#6641=VERTEX_POINT('',#26763);
#6642=VERTEX_POINT('',#26767);
#6643=VERTEX_POINT('',#26771);
#6644=VERTEX_POINT('',#26775);
#6645=VERTEX_POINT('',#26779);
#6646=VERTEX_POINT('',#26783);
#6647=VERTEX_POINT('',#26787);
#6648=VERTEX_POINT('',#26791);
#6649=VERTEX_POINT('',#26802);
#6650=VERTEX_POINT('',#26810);
#6651=VERTEX_POINT('',#26823);
#6652=VERTEX_POINT('',#26830);
#8416=EDGE_CURVE('',#6589,#6590,#4162,.T.);
#8417=EDGE_CURVE('',#6589,#6591,#592,.T.);
#8418=EDGE_CURVE('',#6591,#6592,#1386,.T.);
#8419=EDGE_CURVE('',#6592,#6590,#593,.T.);
#8420=EDGE_CURVE('',#6593,#6594,#4163,.T.);
#8421=EDGE_CURVE('',#6593,#6589,#594,.T.);
#8422=EDGE_CURVE('',#6590,#6594,#595,.T.);
#8423=EDGE_CURVE('',#6595,#6596,#4164,.T.);
#8424=EDGE_CURVE('',#6595,#6593,#596,.T.);
#8425=EDGE_CURVE('',#6594,#6596,#597,.T.);
#8426=EDGE_CURVE('',#6597,#6598,#4165,.T.);
#8427=EDGE_CURVE('',#6597,#6595,#598,.T.);
#8428=EDGE_CURVE('',#6596,#6598,#599,.T.);
#8429=EDGE_CURVE('',#6599,#6600,#4166,.T.);
#8430=EDGE_CURVE('',#6599,#6597,#600,.T.);
#8431=EDGE_CURVE('',#6598,#6600,#601,.T.);
#8432=EDGE_CURVE('',#6601,#6602,#4167,.T.);
#8433=EDGE_CURVE('',#6601,#6603,#602,.T.);
#8434=EDGE_CURVE('',#6602,#6603,#1387,.T.);
#8435=EDGE_CURVE('',#6604,#6605,#4168,.T.);
#8436=EDGE_CURVE('',#6604,#6601,#603,.T.);
#8437=EDGE_CURVE('',#6606,#6602,#1388,.T.);
#8438=EDGE_CURVE('',#6605,#6606,#604,.T.);
#8439=EDGE_CURVE('',#6607,#6608,#4169,.T.);
#8440=EDGE_CURVE('',#6607,#6604,#605,.T.);
#8441=EDGE_CURVE('',#6608,#6605,#606,.T.);
#8442=EDGE_CURVE('',#6609,#6610,#4170,.T.);
#8443=EDGE_CURVE('',#6609,#6607,#607,.T.);
#8444=EDGE_CURVE('',#6610,#6608,#608,.T.);
#8445=EDGE_CURVE('',#6611,#6612,#4171,.T.);
#8446=EDGE_CURVE('',#6611,#6609,#609,.T.);
#8447=EDGE_CURVE('',#6612,#6610,#610,.T.);
#8448=EDGE_CURVE('',#6603,#6613,#611,.T.);
#8449=EDGE_CURVE('',#6614,#6613,#1389,.F.);
#8450=EDGE_CURVE('',#6615,#6614,#1390,.F.);
#8451=EDGE_CURVE('',#6615,#6606,#612,.T.);
#8452=EDGE_CURVE('',#6600,#6615,#613,.T.);
#8453=EDGE_CURVE('',#6616,#6592,#614,.T.);
#8454=EDGE_CURVE('',#6616,#6612,#615,.T.);
#8455=EDGE_CURVE('',#6592,#6617,#1391,.T.);
#8456=EDGE_CURVE('',#6617,#6591,#1392,.T.);
#8457=EDGE_CURVE('',#6591,#6618,#616,.T.);
#8458=EDGE_CURVE('',#6618,#6616,#1393,.T.);
#8459=EDGE_CURVE('',#6618,#6611,#617,.T.);
#8460=EDGE_CURVE('',#6613,#6599,#618,.T.);
#8461=EDGE_CURVE('',#6619,#6620,#4172,.T.);
#8462=EDGE_CURVE('',#6620,#6619,#1394,.T.);
#8463=EDGE_CURVE('',#6620,#6621,#4173,.T.);
#8464=EDGE_CURVE('',#6621,#6620,#1395,.T.);
#8465=EDGE_CURVE('',#6621,#6622,#4174,.T.);
#8466=EDGE_CURVE('',#6622,#6621,#1396,.T.);
#8467=EDGE_CURVE('',#6622,#6623,#4175,.T.);
#8468=EDGE_CURVE('',#6623,#6622,#1397,.T.);
#8469=EDGE_CURVE('',#6623,#6624,#4176,.T.);
#8470=EDGE_CURVE('',#6624,#6623,#1398,.T.);
#8471=EDGE_CURVE('',#6624,#6619,#4177,.T.);
#8472=EDGE_CURVE('',#6619,#6624,#1399,.T.);
#8473=EDGE_CURVE('',#6625,#6626,#4178,.T.);
#8474=EDGE_CURVE('',#6627,#6626,#1400,.T.);
#8475=EDGE_CURVE('',#6621,#6627,#118,.T.);
#8476=EDGE_CURVE('',#6628,#6620,#119,.T.);
#8477=EDGE_CURVE('',#6629,#6628,#1401,.T.);
#8478=EDGE_CURVE('',#6620,#6629,#120,.T.);
#8479=EDGE_CURVE('',#6630,#6619,#121,.T.);
#8480=EDGE_CURVE('',#6631,#6630,#1402,.T.);
#8481=EDGE_CURVE('',#6619,#6631,#122,.T.);
#8482=EDGE_CURVE('',#6632,#6624,#123,.T.);
#8483=EDGE_CURVE('',#6633,#6632,#1403,.T.);
#8484=EDGE_CURVE('',#6624,#6633,#124,.T.);
#8485=EDGE_CURVE('',#6634,#6623,#125,.T.);
#8486=EDGE_CURVE('',#6635,#6634,#1404,.T.);
#8487=EDGE_CURVE('',#6623,#6635,#126,.T.);
#8488=EDGE_CURVE('',#6636,#6622,#127,.T.);
#8489=EDGE_CURVE('',#6637,#6636,#1405,.T.);
#8490=EDGE_CURVE('',#6622,#6637,#128,.T.);
#8491=EDGE_CURVE('',#6638,#6621,#129,.T.);
#8492=EDGE_CURVE('',#6626,#6638,#1406,.T.);
#8493=EDGE_CURVE('',#6639,#6622,#4179,.T.);
#8494=EDGE_CURVE('',#6640,#6639,#4180,.T.);
#8495=EDGE_CURVE('',#6640,#6621,#4181,.T.);
#8496=EDGE_CURVE('',#6621,#6641,#4182,.T.);
#8497=EDGE_CURVE('',#6641,#6638,#4183,.T.);
#8498=EDGE_CURVE('',#6642,#6623,#4184,.T.);
#8499=EDGE_CURVE('',#6639,#6642,#4185,.T.);
#8500=EDGE_CURVE('',#6635,#6643,#4186,.T.);
#8501=EDGE_CURVE('',#6623,#6643,#4187,.T.);
#8502=EDGE_CURVE('',#6622,#6644,#4188,.T.);
#8503=EDGE_CURVE('',#6644,#6636,#4189,.T.);
#8504=EDGE_CURVE('',#6645,#6640,#4190,.T.);
#8505=EDGE_CURVE('',#6645,#6620,#4191,.T.);
#8506=EDGE_CURVE('',#6620,#6646,#4192,.T.);
#8507=EDGE_CURVE('',#6646,#6628,#4193,.T.);
#8508=EDGE_CURVE('',#6647,#6624,#4194,.T.);
#8509=EDGE_CURVE('',#6642,#6647,#4195,.T.);
#8510=EDGE_CURVE('',#6633,#6648,#4196,.T.);
#8511=EDGE_CURVE('',#6624,#6648,#4197,.T.);
#8512=EDGE_CURVE('',#6643,#6634,#4198,.T.);
#8513=EDGE_CURVE('',#6637,#6644,#4199,.T.);
#8514=EDGE_CURVE('',#6648,#6632,#4200,.T.);
#8515=EDGE_CURVE('',#6649,#6630,#4201,.T.);
#8516=EDGE_CURVE('',#6631,#6649,#4202,.T.);
#8517=EDGE_CURVE('',#6629,#6646,#4203,.T.);
#8518=EDGE_CURVE('',#6627,#6641,#4204,.T.);
#8519=EDGE_CURVE('',#6650,#6619,#4205,.T.);
#8520=EDGE_CURVE('',#6647,#6650,#4206,.T.);
#8521=EDGE_CURVE('',#6619,#6649,#4207,.T.);
#8522=EDGE_CURVE('',#6650,#6645,#4208,.T.);
#8523=EDGE_CURVE('',#6651,#6651,#1407,.T.);
#8524=EDGE_CURVE('',#6617,#6651,#4209,.T.);
#8525=EDGE_CURVE('',#6613,#6615,#1408,.F.);
#8526=EDGE_CURVE('',#6652,#6652,#1409,.T.);
#8527=EDGE_CURVE('',#6652,#6614,#4210,.T.);
#11601=ORIENTED_EDGE('',*,*,#8416,.F.);
#11602=ORIENTED_EDGE('',*,*,#8417,.T.);
#11603=ORIENTED_EDGE('',*,*,#8418,.T.);
#11604=ORIENTED_EDGE('',*,*,#8419,.T.);
#11605=ORIENTED_EDGE('',*,*,#8420,.F.);
#11606=ORIENTED_EDGE('',*,*,#8421,.T.);
#11607=ORIENTED_EDGE('',*,*,#8416,.T.);
#11608=ORIENTED_EDGE('',*,*,#8422,.T.);
#11609=ORIENTED_EDGE('',*,*,#8423,.F.);
#11610=ORIENTED_EDGE('',*,*,#8424,.T.);
#11611=ORIENTED_EDGE('',*,*,#8420,.T.);
#11612=ORIENTED_EDGE('',*,*,#8425,.T.);
#11613=ORIENTED_EDGE('',*,*,#8426,.F.);
#11614=ORIENTED_EDGE('',*,*,#8427,.T.);
#11615=ORIENTED_EDGE('',*,*,#8423,.T.);
#11616=ORIENTED_EDGE('',*,*,#8428,.T.);
#11617=ORIENTED_EDGE('',*,*,#8429,.F.);
#11618=ORIENTED_EDGE('',*,*,#8430,.T.);
#11619=ORIENTED_EDGE('',*,*,#8426,.T.);
#11620=ORIENTED_EDGE('',*,*,#8431,.T.);
#11621=ORIENTED_EDGE('',*,*,#8432,.F.);
#11622=ORIENTED_EDGE('',*,*,#8433,.T.);
#11623=ORIENTED_EDGE('',*,*,#8434,.F.);
#11624=ORIENTED_EDGE('',*,*,#8435,.F.);
#11625=ORIENTED_EDGE('',*,*,#8436,.T.);
#11626=ORIENTED_EDGE('',*,*,#8432,.T.);
#11627=ORIENTED_EDGE('',*,*,#8437,.F.);
#11628=ORIENTED_EDGE('',*,*,#8438,.F.);
#11629=ORIENTED_EDGE('',*,*,#8439,.F.);
#11630=ORIENTED_EDGE('',*,*,#8440,.T.);
#11631=ORIENTED_EDGE('',*,*,#8435,.T.);
#11632=ORIENTED_EDGE('',*,*,#8441,.F.);
#11633=ORIENTED_EDGE('',*,*,#8442,.F.);
#11634=ORIENTED_EDGE('',*,*,#8443,.T.);
#11635=ORIENTED_EDGE('',*,*,#8439,.T.);
#11636=ORIENTED_EDGE('',*,*,#8444,.F.);
#11637=ORIENTED_EDGE('',*,*,#8445,.F.);
#11638=ORIENTED_EDGE('',*,*,#8446,.T.);
#11639=ORIENTED_EDGE('',*,*,#8442,.T.);
#11640=ORIENTED_EDGE('',*,*,#8447,.F.);
#11641=ORIENTED_EDGE('',*,*,#8437,.T.);
#11642=ORIENTED_EDGE('',*,*,#8434,.T.);
#11643=ORIENTED_EDGE('',*,*,#8448,.T.);
#11644=ORIENTED_EDGE('',*,*,#8449,.F.);
#11645=ORIENTED_EDGE('',*,*,#8450,.F.);
#11646=ORIENTED_EDGE('',*,*,#8451,.T.);
#11647=ORIENTED_EDGE('',*,*,#8451,.F.);
#11648=ORIENTED_EDGE('',*,*,#8452,.F.);
#11649=ORIENTED_EDGE('',*,*,#8431,.F.);
#11650=ORIENTED_EDGE('',*,*,#8428,.F.);
#11651=ORIENTED_EDGE('',*,*,#8425,.F.);
#11652=ORIENTED_EDGE('',*,*,#8422,.F.);
#11653=ORIENTED_EDGE('',*,*,#8419,.F.);
#11654=ORIENTED_EDGE('',*,*,#8453,.F.);
#11655=ORIENTED_EDGE('',*,*,#8454,.T.);
#11656=ORIENTED_EDGE('',*,*,#8447,.T.);
#11657=ORIENTED_EDGE('',*,*,#8444,.T.);
#11658=ORIENTED_EDGE('',*,*,#8441,.T.);
#11659=ORIENTED_EDGE('',*,*,#8438,.T.);
#11660=ORIENTED_EDGE('',*,*,#8455,.T.);
#11661=ORIENTED_EDGE('',*,*,#8456,.T.);
#11662=ORIENTED_EDGE('',*,*,#8457,.T.);
#11663=ORIENTED_EDGE('',*,*,#8458,.T.);
#11664=ORIENTED_EDGE('',*,*,#8453,.T.);
#11665=ORIENTED_EDGE('',*,*,#8445,.T.);
#11666=ORIENTED_EDGE('',*,*,#8454,.F.);
#11667=ORIENTED_EDGE('',*,*,#8458,.F.);
#11668=ORIENTED_EDGE('',*,*,#8459,.T.);
#11669=ORIENTED_EDGE('',*,*,#8448,.F.);
#11670=ORIENTED_EDGE('',*,*,#8433,.F.);
#11671=ORIENTED_EDGE('',*,*,#8436,.F.);
#11672=ORIENTED_EDGE('',*,*,#8440,.F.);
#11673=ORIENTED_EDGE('',*,*,#8443,.F.);
#11674=ORIENTED_EDGE('',*,*,#8446,.F.);
#11675=ORIENTED_EDGE('',*,*,#8459,.F.);
#11676=ORIENTED_EDGE('',*,*,#8457,.F.);
#11677=ORIENTED_EDGE('',*,*,#8417,.F.);
#11678=ORIENTED_EDGE('',*,*,#8421,.F.);
#11679=ORIENTED_EDGE('',*,*,#8424,.F.);
#11680=ORIENTED_EDGE('',*,*,#8427,.F.);
#11681=ORIENTED_EDGE('',*,*,#8430,.F.);
#11682=ORIENTED_EDGE('',*,*,#8460,.F.);
#11683=ORIENTED_EDGE('',*,*,#8461,.F.);
#11684=ORIENTED_EDGE('',*,*,#8462,.F.);
#11685=ORIENTED_EDGE('',*,*,#8463,.F.);
#11686=ORIENTED_EDGE('',*,*,#8464,.F.);
#11687=ORIENTED_EDGE('',*,*,#8465,.F.);
#11688=ORIENTED_EDGE('',*,*,#8466,.F.);
#11689=ORIENTED_EDGE('',*,*,#8467,.F.);
#11690=ORIENTED_EDGE('',*,*,#8468,.F.);
#11691=ORIENTED_EDGE('',*,*,#8469,.F.);
#11692=ORIENTED_EDGE('',*,*,#8470,.F.);
#11693=ORIENTED_EDGE('',*,*,#8471,.F.);
#11694=ORIENTED_EDGE('',*,*,#8472,.F.);
#11695=ORIENTED_EDGE('',*,*,#8473,.T.);
#11696=ORIENTED_EDGE('',*,*,#8474,.F.);
#11697=ORIENTED_EDGE('',*,*,#8475,.F.);
#11698=ORIENTED_EDGE('',*,*,#8464,.T.);
#11699=ORIENTED_EDGE('',*,*,#8476,.F.);
#11700=ORIENTED_EDGE('',*,*,#8477,.F.);
#11701=ORIENTED_EDGE('',*,*,#8478,.F.);
#11702=ORIENTED_EDGE('',*,*,#8462,.T.);
#11703=ORIENTED_EDGE('',*,*,#8479,.F.);
#11704=ORIENTED_EDGE('',*,*,#8480,.F.);
#11705=ORIENTED_EDGE('',*,*,#8481,.F.);
#11706=ORIENTED_EDGE('',*,*,#8472,.T.);
#11707=ORIENTED_EDGE('',*,*,#8482,.F.);
#11708=ORIENTED_EDGE('',*,*,#8483,.F.);
#11709=ORIENTED_EDGE('',*,*,#8484,.F.);
#11710=ORIENTED_EDGE('',*,*,#8470,.T.);
#11711=ORIENTED_EDGE('',*,*,#8485,.F.);
#11712=ORIENTED_EDGE('',*,*,#8486,.F.);
#11713=ORIENTED_EDGE('',*,*,#8487,.F.);
#11714=ORIENTED_EDGE('',*,*,#8468,.T.);
#11715=ORIENTED_EDGE('',*,*,#8488,.F.);
#11716=ORIENTED_EDGE('',*,*,#8489,.F.);
#11717=ORIENTED_EDGE('',*,*,#8490,.F.);
#11718=ORIENTED_EDGE('',*,*,#8466,.T.);
#11719=ORIENTED_EDGE('',*,*,#8491,.F.);
#11720=ORIENTED_EDGE('',*,*,#8492,.F.);
#11721=ORIENTED_EDGE('',*,*,#8473,.F.);
#11722=ORIENTED_EDGE('',*,*,#8465,.T.);
#11723=ORIENTED_EDGE('',*,*,#8493,.F.);
#11724=ORIENTED_EDGE('',*,*,#8494,.F.);
#11725=ORIENTED_EDGE('',*,*,#8495,.T.);
#11726=ORIENTED_EDGE('',*,*,#8491,.T.);
#11727=ORIENTED_EDGE('',*,*,#8496,.T.);
#11728=ORIENTED_EDGE('',*,*,#8497,.T.);
#11729=ORIENTED_EDGE('',*,*,#8467,.T.);
#11730=ORIENTED_EDGE('',*,*,#8498,.F.);
#11731=ORIENTED_EDGE('',*,*,#8499,.F.);
#11732=ORIENTED_EDGE('',*,*,#8493,.T.);
#11733=ORIENTED_EDGE('',*,*,#8487,.T.);
#11734=ORIENTED_EDGE('',*,*,#8500,.T.);
#11735=ORIENTED_EDGE('',*,*,#8501,.F.);
#11736=ORIENTED_EDGE('',*,*,#8488,.T.);
#11737=ORIENTED_EDGE('',*,*,#8502,.T.);
#11738=ORIENTED_EDGE('',*,*,#8503,.T.);
#11739=ORIENTED_EDGE('',*,*,#8463,.T.);
#11740=ORIENTED_EDGE('',*,*,#8495,.F.);
#11741=ORIENTED_EDGE('',*,*,#8504,.F.);
#11742=ORIENTED_EDGE('',*,*,#8505,.T.);
#11743=ORIENTED_EDGE('',*,*,#8476,.T.);
#11744=ORIENTED_EDGE('',*,*,#8506,.T.);
#11745=ORIENTED_EDGE('',*,*,#8507,.T.);
#11746=ORIENTED_EDGE('',*,*,#8469,.T.);
#11747=ORIENTED_EDGE('',*,*,#8508,.F.);
#11748=ORIENTED_EDGE('',*,*,#8509,.F.);
#11749=ORIENTED_EDGE('',*,*,#8498,.T.);
#11750=ORIENTED_EDGE('',*,*,#8484,.T.);
#11751=ORIENTED_EDGE('',*,*,#8510,.T.);
#11752=ORIENTED_EDGE('',*,*,#8511,.F.);
#11753=ORIENTED_EDGE('',*,*,#8485,.T.);
#11754=ORIENTED_EDGE('',*,*,#8501,.T.);
#11755=ORIENTED_EDGE('',*,*,#8512,.T.);
#11756=ORIENTED_EDGE('',*,*,#8489,.T.);
#11757=ORIENTED_EDGE('',*,*,#8503,.F.);
#11758=ORIENTED_EDGE('',*,*,#8513,.F.);
#11759=ORIENTED_EDGE('',*,*,#8486,.T.);
#11760=ORIENTED_EDGE('',*,*,#8512,.F.);
#11761=ORIENTED_EDGE('',*,*,#8500,.F.);
#11762=ORIENTED_EDGE('',*,*,#8483,.T.);
#11763=ORIENTED_EDGE('',*,*,#8514,.F.);
#11764=ORIENTED_EDGE('',*,*,#8510,.F.);
#11765=ORIENTED_EDGE('',*,*,#8480,.T.);
#11766=ORIENTED_EDGE('',*,*,#8515,.F.);
#11767=ORIENTED_EDGE('',*,*,#8516,.F.);
#11768=ORIENTED_EDGE('',*,*,#8477,.T.);
#11769=ORIENTED_EDGE('',*,*,#8507,.F.);
#11770=ORIENTED_EDGE('',*,*,#8517,.F.);
#11771=ORIENTED_EDGE('',*,*,#8474,.T.);
#11772=ORIENTED_EDGE('',*,*,#8492,.T.);
#11773=ORIENTED_EDGE('',*,*,#8497,.F.);
#11774=ORIENTED_EDGE('',*,*,#8518,.F.);
#11775=ORIENTED_EDGE('',*,*,#8471,.T.);
#11776=ORIENTED_EDGE('',*,*,#8519,.F.);
#11777=ORIENTED_EDGE('',*,*,#8520,.F.);
#11778=ORIENTED_EDGE('',*,*,#8508,.T.);
#11779=ORIENTED_EDGE('',*,*,#8481,.T.);
#11780=ORIENTED_EDGE('',*,*,#8516,.T.);
#11781=ORIENTED_EDGE('',*,*,#8521,.F.);
#11782=ORIENTED_EDGE('',*,*,#8482,.T.);
#11783=ORIENTED_EDGE('',*,*,#8511,.T.);
#11784=ORIENTED_EDGE('',*,*,#8514,.T.);
#11785=ORIENTED_EDGE('',*,*,#8479,.T.);
#11786=ORIENTED_EDGE('',*,*,#8521,.T.);
#11787=ORIENTED_EDGE('',*,*,#8515,.T.);
#11788=ORIENTED_EDGE('',*,*,#8461,.T.);
#11789=ORIENTED_EDGE('',*,*,#8505,.F.);
#11790=ORIENTED_EDGE('',*,*,#8522,.F.);
#11791=ORIENTED_EDGE('',*,*,#8519,.T.);
#11792=ORIENTED_EDGE('',*,*,#8490,.T.);
#11793=ORIENTED_EDGE('',*,*,#8513,.T.);
#11794=ORIENTED_EDGE('',*,*,#8502,.F.);
#11795=ORIENTED_EDGE('',*,*,#8475,.T.);
#11796=ORIENTED_EDGE('',*,*,#8518,.T.);
#11797=ORIENTED_EDGE('',*,*,#8496,.F.);
#11798=ORIENTED_EDGE('',*,*,#8478,.T.);
#11799=ORIENTED_EDGE('',*,*,#8517,.T.);
#11800=ORIENTED_EDGE('',*,*,#8506,.F.);
#11801=ORIENTED_EDGE('',*,*,#8523,.F.);
#11802=ORIENTED_EDGE('',*,*,#8455,.F.);
#11803=ORIENTED_EDGE('',*,*,#8418,.F.);
#11804=ORIENTED_EDGE('',*,*,#8456,.F.);
#11805=ORIENTED_EDGE('',*,*,#8524,.T.);
#11806=ORIENTED_EDGE('',*,*,#8523,.T.);
#11807=ORIENTED_EDGE('',*,*,#8524,.F.);
#11808=ORIENTED_EDGE('',*,*,#8429,.T.);
#11809=ORIENTED_EDGE('',*,*,#8452,.T.);
#11810=ORIENTED_EDGE('',*,*,#8525,.F.);
#11811=ORIENTED_EDGE('',*,*,#8460,.T.);
#11812=ORIENTED_EDGE('',*,*,#8526,.F.);
#11813=ORIENTED_EDGE('',*,*,#8527,.T.);
#11814=ORIENTED_EDGE('',*,*,#8449,.T.);
#11815=ORIENTED_EDGE('',*,*,#8525,.T.);
#11816=ORIENTED_EDGE('',*,*,#8450,.T.);
#11817=ORIENTED_EDGE('',*,*,#8527,.F.);
#11818=ORIENTED_EDGE('',*,*,#8526,.T.);
#11819=ORIENTED_EDGE('',*,*,#8509,.T.);
#11820=ORIENTED_EDGE('',*,*,#8520,.T.);
#11821=ORIENTED_EDGE('',*,*,#8522,.T.);
#11822=ORIENTED_EDGE('',*,*,#8504,.T.);
#11823=ORIENTED_EDGE('',*,*,#8494,.T.);
#11824=ORIENTED_EDGE('',*,*,#8499,.T.);
#14999=PLANE('',#16923);
#15000=PLANE('',#16926);
#15001=PLANE('',#16931);
#15002=PLANE('',#16933);
#15003=PLANE('',#16935);
#15004=PLANE('',#16937);
#15005=PLANE('',#16939);
#15006=PLANE('',#16941);
#15007=PLANE('',#16951);
#15008=PLANE('',#16952);
#15009=PLANE('',#16953);
#15010=PLANE('',#16954);
#15011=PLANE('',#16955);
#15012=PLANE('',#16956);
#15013=PLANE('',#16957);
#15014=PLANE('',#16958);
#15015=PLANE('',#16959);
#15016=PLANE('',#16960);
#15017=PLANE('',#16961);
#15018=PLANE('',#16962);
#15019=PLANE('',#16963);
#15020=PLANE('',#16964);
#15021=PLANE('',#16965);
#15022=PLANE('',#16966);
#15023=PLANE('',#16967);
#15024=PLANE('',#16968);
#15025=PLANE('',#16969);
#15026=PLANE('',#16970);
#15027=PLANE('',#16971);
#15028=PLANE('',#16972);
#15029=PLANE('',#16973);
#15030=PLANE('',#16974);
#15031=PLANE('',#16975);
#15032=PLANE('',#16982);
#15643=ADVANCED_FACE('',(#2100),#930,.T.);
#15644=ADVANCED_FACE('',(#2101),#931,.T.);
#15645=ADVANCED_FACE('',(#2102),#932,.T.);
#15646=ADVANCED_FACE('',(#2103),#933,.T.);
#15647=ADVANCED_FACE('',(#2104),#934,.T.);
#15648=ADVANCED_FACE('',(#2105),#935,.T.);
#15649=ADVANCED_FACE('',(#2106),#936,.T.);
#15650=ADVANCED_FACE('',(#2107),#937,.T.);
#15651=ADVANCED_FACE('',(#2108),#938,.T.);
#15652=ADVANCED_FACE('',(#2109),#939,.T.);
#15653=ADVANCED_FACE('',(#2110),#14999,.F.);
#15654=ADVANCED_FACE('',(#2111),#499,.F.);
#15655=ADVANCED_FACE('',(#2112),#15000,.T.);
#15656=ADVANCED_FACE('',(#2113),#940,.T.);
#15657=ADVANCED_FACE('',(#2114),#500,.F.);
#15658=ADVANCED_FACE('',(#2115),#15001,.F.);
#15659=ADVANCED_FACE('',(#2116),#15002,.F.);
#15660=ADVANCED_FACE('',(#2117),#15003,.F.);
#15661=ADVANCED_FACE('',(#2118),#15004,.F.);
#15662=ADVANCED_FACE('',(#2119),#15005,.F.);
#15663=ADVANCED_FACE('',(#2120),#15006,.F.);
#15664=ADVANCED_FACE('',(#2121),#1743,.F.);
#15665=ADVANCED_FACE('',(#2122),#15007,.F.);
#15666=ADVANCED_FACE('',(#2123),#15008,.F.);
#15667=ADVANCED_FACE('',(#2124),#15009,.F.);
#15668=ADVANCED_FACE('',(#2125),#15010,.F.);
#15669=ADVANCED_FACE('',(#2126),#15011,.F.);
#15670=ADVANCED_FACE('',(#2127),#15012,.F.);
#15671=ADVANCED_FACE('',(#2128),#15013,.F.);
#15672=ADVANCED_FACE('',(#2129),#15014,.F.);
#15673=ADVANCED_FACE('',(#2130),#15015,.F.);
#15674=ADVANCED_FACE('',(#2131),#15016,.F.);
#15675=ADVANCED_FACE('',(#2132),#15017,.F.);
#15676=ADVANCED_FACE('',(#2133),#15018,.F.);
#15677=ADVANCED_FACE('',(#2134),#15019,.F.);
#15678=ADVANCED_FACE('',(#2135),#15020,.F.);
#15679=ADVANCED_FACE('',(#2136),#15021,.F.);
#15680=ADVANCED_FACE('',(#2137),#15022,.F.);
#15681=ADVANCED_FACE('',(#2138),#15023,.F.);
#15682=ADVANCED_FACE('',(#2139),#15024,.F.);
#15683=ADVANCED_FACE('',(#2140),#15025,.F.);
#15684=ADVANCED_FACE('',(#2141),#15026,.F.);
#15685=ADVANCED_FACE('',(#2142),#15027,.F.);
#15686=ADVANCED_FACE('',(#2143),#15028,.F.);
#15687=ADVANCED_FACE('',(#2144),#15029,.F.);
#15688=ADVANCED_FACE('',(#2145),#15030,.F.);
#15689=ADVANCED_FACE('',(#2146),#15031,.T.);
#15690=ADVANCED_FACE('',(#2147),#1744,.T.);
#15691=ADVANCED_FACE('',(#2148),#941,.T.);
#15692=ADVANCED_FACE('',(#2149),#1745,.T.);
#15693=ADVANCED_FACE('',(#2150,#1187),#15032,.T.);
#16241=CLOSED_SHELL('',(#15643,#15644,#15645,#15646,#15647,#15648,#15649,
#15650,#15651,#15652,#15653,#15654,#15655,#15656,#15657,#15658,#15659,#15660,
#15661,#15662,#15663,#15664,#15665,#15666,#15667,#15668,#15669,#15670,#15671,
#15672,#15673,#15674,#15675,#15676,#15677,#15678,#15679,#15680,#15681,#15682,
#15683,#15684,#15685,#15686,#15687,#15688,#15689,#15690,#15691,#15692,#15693));
#16909=AXIS2_PLACEMENT_3D('',#25793,#19325,#19326);
#16910=AXIS2_PLACEMENT_3D('',#25794,#19327,#19328);
#16911=AXIS2_PLACEMENT_3D('',#25810,#19330,#19331);
#16912=AXIS2_PLACEMENT_3D('',#25818,#19332,#19333);
#16913=AXIS2_PLACEMENT_3D('',#25866,#19335,#19336);
#16914=AXIS2_PLACEMENT_3D('',#25914,#19338,#19339);
#16915=AXIS2_PLACEMENT_3D('',#25968,#19341,#19342);
#16916=AXIS2_PLACEMENT_3D('',#26016,#19344,#19345);
#16917=AXIS2_PLACEMENT_3D('',#26025,#19347,#19348);
#16918=AXIS2_PLACEMENT_3D('',#26026,#19349,#19350);
#16919=AXIS2_PLACEMENT_3D('',#26041,#19352,#19353);
#16920=AXIS2_PLACEMENT_3D('',#26051,#19354,#19355);
#16921=AXIS2_PLACEMENT_3D('',#26076,#19357,#19358);
#16922=AXIS2_PLACEMENT_3D('',#26101,#19360,#19361);
#16923=AXIS2_PLACEMENT_3D('',#26125,#19363,#19364);
#16924=AXIS2_PLACEMENT_3D('',#26180,#19365,#19366);
#16925=AXIS2_PLACEMENT_3D('',#26182,#19367,#19368);
#16926=AXIS2_PLACEMENT_3D('',#26453,#19369,#19370);
#16927=AXIS2_PLACEMENT_3D('',#26455,#19371,#19372);
#16928=AXIS2_PLACEMENT_3D('',#26456,#19373,#19374);
#16929=AXIS2_PLACEMENT_3D('',#26513,#19375,#19376);
#16930=AXIS2_PLACEMENT_3D('',#26514,#19377,#19378);
#16931=AXIS2_PLACEMENT_3D('',#26673,#19379,#19380);
#16932=AXIS2_PLACEMENT_3D('',#26677,#19382,#19383);
#16933=AXIS2_PLACEMENT_3D('',#26678,#19384,#19385);
#16934=AXIS2_PLACEMENT_3D('',#26681,#19387,#19388);
#16935=AXIS2_PLACEMENT_3D('',#26682,#19389,#19390);
#16936=AXIS2_PLACEMENT_3D('',#26685,#19392,#19393);
#16937=AXIS2_PLACEMENT_3D('',#26686,#19394,#19395);
#16938=AXIS2_PLACEMENT_3D('',#26689,#19397,#19398);
#16939=AXIS2_PLACEMENT_3D('',#26690,#19399,#19400);
#16940=AXIS2_PLACEMENT_3D('',#26693,#19402,#19403);
#16941=AXIS2_PLACEMENT_3D('',#26694,#19404,#19405);
#16942=AXIS2_PLACEMENT_3D('',#26696,#19407,#19408);
#16943=AXIS2_PLACEMENT_3D('',#26697,#19409,#19410);
#16944=AXIS2_PLACEMENT_3D('',#26702,#19412,#19413);
#16945=AXIS2_PLACEMENT_3D('',#26711,#19414,#19415);
#16946=AXIS2_PLACEMENT_3D('',#26720,#19416,#19417);
#16947=AXIS2_PLACEMENT_3D('',#26729,#19418,#19419);
#16948=AXIS2_PLACEMENT_3D('',#26738,#19420,#19421);
#16949=AXIS2_PLACEMENT_3D('',#26747,#19422,#19423);
#16950=AXIS2_PLACEMENT_3D('',#26755,#19424,#19425);
#16951=AXIS2_PLACEMENT_3D('',#26756,#19426,#19427);
#16952=AXIS2_PLACEMENT_3D('',#26762,#19431,#19432);
#16953=AXIS2_PLACEMENT_3D('',#26766,#19435,#19436);
#16954=AXIS2_PLACEMENT_3D('',#26770,#19439,#19440);
#16955=AXIS2_PLACEMENT_3D('',#26774,#19443,#19444);
#16956=AXIS2_PLACEMENT_3D('',#26778,#19447,#19448);
#16957=AXIS2_PLACEMENT_3D('',#26782,#19451,#19452);
#16958=AXIS2_PLACEMENT_3D('',#26786,#19455,#19456);
#16959=AXIS2_PLACEMENT_3D('',#26790,#19459,#19460);
#16960=AXIS2_PLACEMENT_3D('',#26794,#19463,#19464);
#16961=AXIS2_PLACEMENT_3D('',#26796,#19466,#19467);
#16962=AXIS2_PLACEMENT_3D('',#26798,#19469,#19470);
#16963=AXIS2_PLACEMENT_3D('',#26799,#19471,#19472);
#16964=AXIS2_PLACEMENT_3D('',#26801,#19474,#19475);
#16965=AXIS2_PLACEMENT_3D('',#26805,#19478,#19479);
#16966=AXIS2_PLACEMENT_3D('',#26807,#19481,#19482);
#16967=AXIS2_PLACEMENT_3D('',#26809,#19484,#19485);
#16968=AXIS2_PLACEMENT_3D('',#26813,#19488,#19489);
#16969=AXIS2_PLACEMENT_3D('',#26815,#19491,#19492);
#16970=AXIS2_PLACEMENT_3D('',#26816,#19493,#19494);
#16971=AXIS2_PLACEMENT_3D('',#26817,#19495,#19496);
#16972=AXIS2_PLACEMENT_3D('',#26819,#19498,#19499);
#16973=AXIS2_PLACEMENT_3D('',#26820,#19500,#19501);
#16974=AXIS2_PLACEMENT_3D('',#26821,#19502,#19503);
#16975=AXIS2_PLACEMENT_3D('',#26822,#19504,#19505);
#16976=AXIS2_PLACEMENT_3D('',#26824,#19506,#19507);
#16977=AXIS2_PLACEMENT_3D('',#26825,#19508,#19509);
#16978=AXIS2_PLACEMENT_3D('',#26827,#19511,#19512);
#16979=AXIS2_PLACEMENT_3D('',#26828,#19513,#19514);
#16980=AXIS2_PLACEMENT_3D('',#26829,#19515,#19516);
#16981=AXIS2_PLACEMENT_3D('',#26831,#19517,#19518);
#16982=AXIS2_PLACEMENT_3D('',#26833,#19520,#19521);
#19325=DIRECTION('axis',(0.,0.,1.));
#19326=DIRECTION('refdir',(1.,0.,0.));
#19327=DIRECTION('center_axis',(0.,0.,1.));
#19328=DIRECTION('ref_axis',(1.,0.,0.));
#19329=DIRECTION('',(0.,0.,-1.));
#19330=DIRECTION('center_axis',(0.,0.,1.));
#19331=DIRECTION('ref_axis',(1.,0.,0.));
#19332=DIRECTION('center_axis',(0.,0.,1.));
#19333=DIRECTION('ref_axis',(1.,0.,0.));
#19334=DIRECTION('',(0.,0.,-1.));
#19335=DIRECTION('center_axis',(0.,0.,1.));
#19336=DIRECTION('ref_axis',(1.,0.,0.));
#19337=DIRECTION('',(0.,0.,-1.));
#19338=DIRECTION('center_axis',(0.,0.,1.));
#19339=DIRECTION('ref_axis',(1.,0.,0.));
#19340=DIRECTION('',(0.,0.,-1.));
#19341=DIRECTION('center_axis',(0.,0.,1.));
#19342=DIRECTION('ref_axis',(1.,0.,0.));
#19343=DIRECTION('',(0.,0.,-1.));
#19344=DIRECTION('center_axis',(0.,0.,1.));
#19345=DIRECTION('ref_axis',(1.,3.07677254327731E-16,0.));
#19346=DIRECTION('',(0.,0.,1.));
#19347=DIRECTION('center_axis',(0.,0.,1.));
#19348=DIRECTION('ref_axis',(1.,3.07677254327731E-16,0.));
#19349=DIRECTION('center_axis',(0.,0.,1.));
#19350=DIRECTION('ref_axis',(1.,3.07677254327731E-16,0.));
#19351=DIRECTION('',(0.,0.,1.));
#19352=DIRECTION('center_axis',(0.,0.,1.));
#19353=DIRECTION('ref_axis',(1.,3.07677254327731E-16,0.));
#19354=DIRECTION('center_axis',(0.,0.,1.));
#19355=DIRECTION('ref_axis',(1.,3.07677254327731E-16,0.));
#19356=DIRECTION('',(0.,0.,1.));
#19357=DIRECTION('center_axis',(0.,0.,1.));
#19358=DIRECTION('ref_axis',(1.,3.07677254327731E-16,0.));
#19359=DIRECTION('',(0.,0.,1.));
#19360=DIRECTION('center_axis',(0.,0.,1.));
#19361=DIRECTION('ref_axis',(1.,3.07677254327731E-16,0.));
#19362=DIRECTION('',(0.,0.,1.));
#19363=DIRECTION('center_axis',(0.,0.,1.));
#19364=DIRECTION('ref_axis',(1.,0.,0.));
#19365=DIRECTION('center_axis',(0.,0.,-1.));
#19366=DIRECTION('ref_axis',(1.,0.,0.));
#19367=DIRECTION('center_axis',(0.,0.,-1.));
#19368=DIRECTION('ref_axis',(1.,0.,0.));
#19369=DIRECTION('center_axis',(0.,0.,1.));
#19370=DIRECTION('ref_axis',(1.,0.,0.));
#19371=DIRECTION('center_axis',(0.,0.,1.));
#19372=DIRECTION('ref_axis',(1.,0.,0.));
#19373=DIRECTION('center_axis',(0.,0.,1.));
#19374=DIRECTION('ref_axis',(1.,0.,0.));
#19375=DIRECTION('center_axis',(0.,0.,-1.));
#19376=DIRECTION('ref_axis',(1.,3.07677254327731E-16,0.));
#19377=DIRECTION('center_axis',(0.,0.,1.));
#19378=DIRECTION('ref_axis',(0.889158769900871,0.457598822013749,0.));
#19379=DIRECTION('center_axis',(0.,0.,1.));
#19380=DIRECTION('ref_axis',(1.,0.,0.));
#19381=DIRECTION('',(-1.,2.40370335797945E-16,0.));
#19382=DIRECTION('center_axis',(0.,0.,1.));
#19383=DIRECTION('ref_axis',(1.,0.,0.));
#19384=DIRECTION('center_axis',(0.,0.,1.));
#19385=DIRECTION('ref_axis',(1.,0.,0.));
#19386=DIRECTION('',(-0.5,0.866025403784439,0.));
#19387=DIRECTION('center_axis',(0.,0.,1.));
#19388=DIRECTION('ref_axis',(1.,0.,0.));
#19389=DIRECTION('center_axis',(0.,0.,1.));
#19390=DIRECTION('ref_axis',(1.,0.,0.));
#19391=DIRECTION('',(0.5,0.866025403784439,0.));
#19392=DIRECTION('center_axis',(0.,0.,1.));
#19393=DIRECTION('ref_axis',(1.,0.,0.));
#19394=DIRECTION('center_axis',(0.,0.,1.));
#19395=DIRECTION('ref_axis',(1.,0.,0.));
#19396=DIRECTION('',(1.,-1.20185167898973E-16,0.));
#19397=DIRECTION('center_axis',(0.,0.,1.));
#19398=DIRECTION('ref_axis',(1.,0.,0.));
#19399=DIRECTION('center_axis',(0.,0.,1.));
#19400=DIRECTION('ref_axis',(1.,0.,0.));
#19401=DIRECTION('',(0.5,-0.866025403784439,0.));
#19402=DIRECTION('center_axis',(0.,0.,1.));
#19403=DIRECTION('ref_axis',(1.,0.,0.));
#19404=DIRECTION('center_axis',(0.,0.,1.));
#19405=DIRECTION('ref_axis',(1.,0.,0.));
#19406=DIRECTION('',(-0.5,-0.866025403784439,0.));
#19407=DIRECTION('center_axis',(0.,0.,1.));
#19408=DIRECTION('ref_axis',(1.,0.,0.));
#19409=DIRECTION('center_axis',(0.,0.,1.));
#19410=DIRECTION('ref_axis',(1.,0.,0.));
#19411=DIRECTION('',(-0.854211984955561,-1.04610797316913E-16,0.519924883765223));
#19412=DIRECTION('center_axis',(0.,0.,-1.));
#19413=DIRECTION('ref_axis',(1.,0.,0.));
#19414=DIRECTION('center_axis',(0.,0.,-1.));
#19415=DIRECTION('ref_axis',(1.,0.,0.));
#19416=DIRECTION('center_axis',(0.,0.,-1.));
#19417=DIRECTION('ref_axis',(1.,0.,0.));
#19418=DIRECTION('center_axis',(0.,0.,-1.));
#19419=DIRECTION('ref_axis',(1.,0.,0.));
#19420=DIRECTION('center_axis',(0.,0.,-1.));
#19421=DIRECTION('ref_axis',(1.,0.,0.));
#19422=DIRECTION('center_axis',(0.,0.,-1.));
#19423=DIRECTION('ref_axis',(1.,0.,0.));
#19424=DIRECTION('center_axis',(0.,0.,-1.));
#19425=DIRECTION('ref_axis',(1.,0.,0.));
#19426=DIRECTION('center_axis',(-0.866025403784439,0.5,0.));
#19427=DIRECTION('ref_axis',(0.5,0.866025403784439,0.));
#19428=DIRECTION('',(0.,0.,-1.));
#19429=DIRECTION('',(0.5,0.866025403784439,0.));
#19430=DIRECTION('',(0.,0.,-1.));
#19431=DIRECTION('center_axis',(-0.866025403784439,0.5,0.));
#19432=DIRECTION('ref_axis',(0.5,0.866025403784439,0.));
#19433=DIRECTION('',(0.,0.,-1.));
#19434=DIRECTION('',(0.5,0.866025403784439,0.));
#19435=DIRECTION('center_axis',(1.20185167898973E-16,1.,0.));
#19436=DIRECTION('ref_axis',(1.,-1.20185167898973E-16,0.));
#19437=DIRECTION('',(0.,0.,-1.));
#19438=DIRECTION('',(1.,-1.20185167898973E-16,0.));
#19439=DIRECTION('center_axis',(1.20185167898973E-16,1.,0.));
#19440=DIRECTION('ref_axis',(1.,-1.20185167898973E-16,0.));
#19441=DIRECTION('',(1.,-1.20185167898973E-16,0.));
#19442=DIRECTION('',(0.,0.,-1.));
#19443=DIRECTION('center_axis',(1.20185167898973E-16,1.,0.));
#19444=DIRECTION('ref_axis',(1.,-1.20185167898973E-16,0.));
#19445=DIRECTION('',(0.,0.,-1.));
#19446=DIRECTION('',(1.,-1.20185167898973E-16,0.));
#19447=DIRECTION('center_axis',(-0.866025403784439,-0.5,0.));
#19448=DIRECTION('ref_axis',(-0.5,0.866025403784439,0.));
#19449=DIRECTION('',(-0.5,0.866025403784439,0.));
#19450=DIRECTION('',(0.,0.,-1.));
#19451=DIRECTION('center_axis',(-0.866025403784439,-0.5,0.));
#19452=DIRECTION('ref_axis',(-0.5,0.866025403784439,0.));
#19453=DIRECTION('',(0.,0.,-1.));
#19454=DIRECTION('',(-0.5,0.866025403784439,0.));
#19455=DIRECTION('center_axis',(0.866025403784439,0.5,0.));
#19456=DIRECTION('ref_axis',(0.5,-0.866025403784439,0.));
#19457=DIRECTION('',(0.,0.,-1.));
#19458=DIRECTION('',(0.5,-0.866025403784439,0.));
#19459=DIRECTION('center_axis',(0.866025403784439,0.5,0.));
#19460=DIRECTION('ref_axis',(0.5,-0.866025403784439,0.));
#19461=DIRECTION('',(0.5,-0.866025403784439,0.));
#19462=DIRECTION('',(0.,0.,-1.));
#19463=DIRECTION('center_axis',(0.866025403784439,0.5,0.));
#19464=DIRECTION('ref_axis',(0.5,-0.866025403784439,0.));
#19465=DIRECTION('',(0.5,-0.866025403784439,0.));
#19466=DIRECTION('center_axis',(0.,0.,-1.));
#19467=DIRECTION('ref_axis',(-1.,0.,0.));
#19468=DIRECTION('',(0.5,0.866025403784439,0.));
#19469=DIRECTION('center_axis',(0.,0.,-1.));
#19470=DIRECTION('ref_axis',(-1.,0.,0.));
#19471=DIRECTION('center_axis',(0.,0.,-1.));
#19472=DIRECTION('ref_axis',(-1.,0.,0.));
#19473=DIRECTION('',(-0.5,-0.866025403784439,0.));
#19474=DIRECTION('center_axis',(0.,0.,-1.));
#19475=DIRECTION('ref_axis',(-1.,0.,0.));
#19476=DIRECTION('',(-1.,2.40370335797945E-16,0.));
#19477=DIRECTION('',(-0.5,-0.866025403784439,0.));
#19478=DIRECTION('center_axis',(0.,0.,-1.));
#19479=DIRECTION('ref_axis',(-1.,0.,0.));
#19480=DIRECTION('',(-1.,2.40370335797945E-16,0.));
#19481=DIRECTION('center_axis',(0.,0.,-1.));
#19482=DIRECTION('ref_axis',(-1.,0.,0.));
#19483=DIRECTION('',(-0.5,0.866025403784439,0.));
#19484=DIRECTION('center_axis',(0.866025403784439,-0.5,0.));
#19485=DIRECTION('ref_axis',(-0.5,-0.866025403784439,0.));
#19486=DIRECTION('',(0.,0.,-1.));
#19487=DIRECTION('',(-0.5,-0.866025403784439,0.));
#19488=DIRECTION('center_axis',(0.866025403784439,-0.5,0.));
#19489=DIRECTION('ref_axis',(-0.5,-0.866025403784439,0.));
#19490=DIRECTION('',(0.,0.,-1.));
#19491=DIRECTION('center_axis',(0.866025403784439,-0.5,0.));
#19492=DIRECTION('ref_axis',(-0.5,-0.866025403784439,0.));
#19493=DIRECTION('center_axis',(-2.40370335797945E-16,-1.,0.));
#19494=DIRECTION('ref_axis',(-1.,2.40370335797945E-16,0.));
#19495=DIRECTION('center_axis',(-2.40370335797945E-16,-1.,0.));
#19496=DIRECTION('ref_axis',(-1.,2.40370335797945E-16,0.));
#19497=DIRECTION('',(-1.,2.40370335797945E-16,0.));
#19498=DIRECTION('center_axis',(-0.866025403784439,0.5,0.));
#19499=DIRECTION('ref_axis',(0.5,0.866025403784439,0.));
#19500=DIRECTION('center_axis',(-0.866025403784439,-0.5,0.));
#19501=DIRECTION('ref_axis',(-0.5,0.866025403784439,0.));
#19502=DIRECTION('center_axis',(-2.40370335797945E-16,-1.,0.));
#19503=DIRECTION('ref_axis',(-1.,2.40370335797945E-16,0.));
#19504=DIRECTION('center_axis',(0.,0.,-1.));
#19505=DIRECTION('ref_axis',(-1.,0.,0.));
#19506=DIRECTION('center_axis',(0.,0.,1.));
#19507=DIRECTION('ref_axis',(1.,0.,0.));
#19508=DIRECTION('center_axis',(0.,0.,1.));
#19509=DIRECTION('ref_axis',(1.,0.,0.));
#19510=DIRECTION('',(0.832050294337843,1.01896772969045E-16,-0.554700196225229));
#19511=DIRECTION('center_axis',(0.,0.,1.));
#19512=DIRECTION('ref_axis',(1.,0.,0.));
#19513=DIRECTION('center_axis',(0.,0.,-1.));
#19514=DIRECTION('ref_axis',(1.,0.,0.));
#19515=DIRECTION('center_axis',(0.,0.,-1.));
#19516=DIRECTION('ref_axis',(1.,0.,0.));
#19517=DIRECTION('center_axis',(0.,0.,1.));
#19518=DIRECTION('ref_axis',(1.,0.,0.));
#19519=DIRECTION('',(-0.707106781186548,-8.65956056235494E-17,-0.707106781186547));
#19520=DIRECTION('center_axis',(0.,0.,1.));
#19521=DIRECTION('ref_axis',(1.,0.,0.));
#25793=CARTESIAN_POINT('',(0.,0.,0.));
#25794=CARTESIAN_POINT('Origin',(0.,0.,-0.19));
#25795=CARTESIAN_POINT('',(-0.195529498469593,0.00015768127982491,-0.330479697454243));
#25796=CARTESIAN_POINT('',(-0.195550405894074,0.000204984114986345,-0.34065363587909));
#25797=CARTESIAN_POINT('',(-0.1954,-2.39295984553393E-17,-0.19));
#25798=CARTESIAN_POINT('',(0.0862527678113333,0.175483407289205,-0.353066666666667));
#25799=CARTESIAN_POINT('Ctrl Pts',(-0.195529498469593,0.00015768127982491,
-0.330479697454243));
#25800=CARTESIAN_POINT('Ctrl Pts',(-0.195614985209273,0.0104270003956845,
-0.331066403480209));
#25801=CARTESIAN_POINT('Ctrl Pts',(-0.194873746209122,0.0206833915158047,
-0.331653109506174));
#25802=CARTESIAN_POINT('Ctrl Pts',(-0.193261993352752,0.0308003123059383,
-0.332239815532139));
#25803=CARTESIAN_POINT('Ctrl Pts',(-0.183227156255684,0.0937886616993844,
-0.33589267047895));
#25804=CARTESIAN_POINT('Ctrl Pts',(-0.139448095221308,0.151370643331935,
-0.339545525425761));
#25805=CARTESIAN_POINT('Ctrl Pts',(-0.0814380303326093,0.177933707035516,
-0.343198380372573));
#25806=CARTESIAN_POINT('Ctrl Pts',(-0.0291994446604737,0.201853985036518,
-0.346487809137271));
#25807=CARTESIAN_POINT('Ctrl Pts',(0.034579296332332,0.200620511802275,
-0.349777237901969));
#25808=CARTESIAN_POINT('Ctrl Pts',(0.0863529496556118,0.175584683415657,
-0.353066666666667));
#25809=CARTESIAN_POINT('',(-0.0861525859670515,0.175382131162755,-0.353066666666667));
#25810=CARTESIAN_POINT('Origin',(0.,0.,-0.353066666666667));
#25811=CARTESIAN_POINT('Ctrl Pts',(-0.0861525859670515,0.175382131162755,
-0.353066666666667));
#25812=CARTESIAN_POINT('Ctrl Pts',(-0.143656790266726,0.147134464929317,
-0.349413811719856));
#25813=CARTESIAN_POINT('Ctrl Pts',(-0.185739203174332,0.0886770108875964,
-0.345760956773044));
#25814=CARTESIAN_POINT('Ctrl Pts',(-0.194015268225219,0.0255264096968064,
-0.342108101826233));
#25815=CARTESIAN_POINT('Ctrl Pts',(-0.195113701730712,0.0171448013100274,
-0.341623279843852));
#25816=CARTESIAN_POINT('Ctrl Pts',(-0.195616612964559,0.00868051988020842,
-0.341138457861471));
#25817=CARTESIAN_POINT('Ctrl Pts',(-0.195550405894074,0.000204984114986345,
-0.34065363587909));
#25818=CARTESIAN_POINT('Origin',(0.,0.,-0.19));
#25819=CARTESIAN_POINT('',(-0.195110707760101,-4.72585694041849E-5,-0.260479697454244));
#25820=CARTESIAN_POINT('',(-0.195100849729129,-1.92665112341343E-5,-0.27065363587909));
#25821=CARTESIAN_POINT('',(-0.1954,-2.39295984553393E-17,-0.19));
#25822=CARTESIAN_POINT('Ctrl Pts',(-0.195110707760101,-4.72585694041849E-5,
-0.260479697454244));
#25823=CARTESIAN_POINT('Ctrl Pts',(-0.19503202637266,0.0352043980738878,
-0.262482607132675));
#25824=CARTESIAN_POINT('Ctrl Pts',(-0.185884422793289,0.0704940830525105,
-0.264485516811107));
#25825=CARTESIAN_POINT('Ctrl Pts',(-0.167920692172535,0.100506798190785,
-0.266488426489538));
#25826=CARTESIAN_POINT('Ctrl Pts',(-0.135158904175888,0.155243212988051,
-0.270141281436349));
#25827=CARTESIAN_POINT('Ctrl Pts',(-0.073073335453198,0.192427622718924,
-0.27379413638316));
#25828=CARTESIAN_POINT('Ctrl Pts',(-0.00935407487596699,0.195477079378747,
-0.277446991329971));
#25829=CARTESIAN_POINT('Ctrl Pts',(0.0543651857012641,0.19852653603857,
-0.281099846276782));
#25830=CARTESIAN_POINT('Ctrl Pts',(0.119718138133036,0.167441039627343,
-0.284752701223594));
#25831=CARTESIAN_POINT('Ctrl Pts',(0.157556692003627,0.116082124071139,
-0.288405556170405));
#25832=CARTESIAN_POINT('Ctrl Pts',(0.195395245874219,0.0647232085149348,
-0.292058411117216));
#25833=CARTESIAN_POINT('Ctrl Pts',(0.205719401183631,-0.00690912618624702,
-0.295711266064027));
#25834=CARTESIAN_POINT('Ctrl Pts',(0.183925482710756,-0.0668615165007966,
-0.299364121010839));
#25835=CARTESIAN_POINT('Ctrl Pts',(0.16213156423788,-0.126813906815346,
-0.30301697595765));
#25836=CARTESIAN_POINT('Ctrl Pts',(0.108219571982719,-0.175086352743264,
-0.306669830904461));
#25837=CARTESIAN_POINT('Ctrl Pts',(0.0462326364389881,-0.19015902116139,
-0.310322685851272));
#25838=CARTESIAN_POINT('Ctrl Pts',(-0.0157542991047424,-0.205231689579517,
-0.313975540798083));
#25839=CARTESIAN_POINT('Ctrl Pts',(-0.0858161779370413,-0.187104580487853,
-0.317628395744894));
#25840=CARTESIAN_POINT('Ctrl Pts',(-0.132701810773311,-0.143843667364851,
-0.321281250691706));
#25841=CARTESIAN_POINT('Ctrl Pts',(-0.172056872668009,-0.107531138119007,
-0.324347399612552));
#25842=CARTESIAN_POINT('Ctrl Pts',(-0.195082741383395,-0.0535101870075604,
-0.327413548533398));
#25843=CARTESIAN_POINT('Ctrl Pts',(-0.195529498469593,0.00015768127982491,
-0.330479697454243));
#25844=CARTESIAN_POINT('Ctrl Pts',(-0.195550405894074,0.000204984114986345,
-0.34065363587909));
#25845=CARTESIAN_POINT('Ctrl Pts',(-0.195117780746291,-0.0551777701148348,
-0.33748560291466));
#25846=CARTESIAN_POINT('Ctrl Pts',(-0.170384536859063,-0.111041069974121,
-0.33431756995023));
#25847=CARTESIAN_POINT('Ctrl Pts',(-0.128717685823896,-0.147458271836019,
-0.3311495369858));
#25848=CARTESIAN_POINT('Ctrl Pts',(-0.0806743211775187,-0.189448603838194,
-0.327496682038988));
#25849=CARTESIAN_POINT('Ctrl Pts',(-0.0101178746905964,-0.205585519502686,
-0.323843827092177));
#25850=CARTESIAN_POINT('Ctrl Pts',(0.0514379301081016,-0.188803240428617,
-0.320190972145366));
#25851=CARTESIAN_POINT('Ctrl Pts',(0.1129937349068,-0.172020961354547,-0.316538117198555));
#25852=CARTESIAN_POINT('Ctrl Pts',(0.165548898017274,-0.122319487541918,
-0.312885262251744));
#25853=CARTESIAN_POINT('Ctrl Pts',(0.18568706648142,-0.0617993993866737,
-0.309232407304933));
#25854=CARTESIAN_POINT('Ctrl Pts',(0.205825234945567,-0.00127931123142962,
-0.305579552358121));
#25855=CARTESIAN_POINT('Ctrl Pts',(0.193546408763386,0.0700593912664289,
-0.30192669741131));
#25856=CARTESIAN_POINT('Ctrl Pts',(0.154314767542849,0.120364936306517,
-0.298273842464499));
#25857=CARTESIAN_POINT('Ctrl Pts',(0.115083126322312,0.170670481346605,
-0.294620987517688));
#25858=CARTESIAN_POINT('Ctrl Pts',(0.0488986700634175,0.199942868928924,
-0.290968132570877));
#25859=CARTESIAN_POINT('Ctrl Pts',(-0.0147137545984364,0.195144562135855,
-0.287315277624065));
#25860=CARTESIAN_POINT('Ctrl Pts',(-0.0783261792602905,0.190346255342787,
-0.283662422677254));
#25861=CARTESIAN_POINT('Ctrl Pts',(-0.139366572325104,0.151477254174331,
-0.280009567730443));
#25862=CARTESIAN_POINT('Ctrl Pts',(-0.170614086184577,0.0958638092691071,
-0.276356712783632));
#25863=CARTESIAN_POINT('Ctrl Pts',(-0.186875976058951,0.0669213557782296,
-0.274455687148784));
#25864=CARTESIAN_POINT('Ctrl Pts',(-0.195068794346351,0.0334438550277428,
-0.272554661513937));
#25865=CARTESIAN_POINT('Ctrl Pts',(-0.195100849729129,-1.92665112341343E-5,
-0.27065363587909));
#25866=CARTESIAN_POINT('Origin',(0.,0.,-0.19));
#25867=CARTESIAN_POINT('',(-0.195668453670677,-6.92573205455238E-5,-0.190479697454244));
#25868=CARTESIAN_POINT('',(-0.195637235488324,-9.58052375767378E-5,-0.20065363587909));
#25869=CARTESIAN_POINT('',(-0.1954,-2.39295984553393E-17,-0.19));
#25870=CARTESIAN_POINT('Ctrl Pts',(-0.195668453670677,-6.92573205455238E-5,
-0.190479697454244));
#25871=CARTESIAN_POINT('Ctrl Pts',(-0.195389991269708,0.0596676372169134,
-0.193898810785141));
#25872=CARTESIAN_POINT('Ctrl Pts',(-0.165981871671571,0.119642236981856,
-0.197317924116039));
#25873=CARTESIAN_POINT('Ctrl Pts',(-0.118451210421177,0.155782728391626,
-0.200737037446937));
#25874=CARTESIAN_POINT('Ctrl Pts',(-0.0676711998538972,0.194393900368106,
-0.204389892393748));
#25875=CARTESIAN_POINT('Ctrl Pts',(0.00379387942481049,0.205800821502601,
-0.208042747340559));
#25876=CARTESIAN_POINT('Ctrl Pts',(0.0640703860629371,0.18491600234246,
-0.21169560228737));
#25877=CARTESIAN_POINT('Ctrl Pts',(0.124346892701064,0.164031183182318,
-0.215348457234181));
#25878=CARTESIAN_POINT('Ctrl Pts',(0.17343482669861,0.110854623727541,-0.219001312180993));
#25879=CARTESIAN_POINT('Ctrl Pts',(0.189440826068912,0.0491031668771414,
-0.222654167127804));
#25880=CARTESIAN_POINT('Ctrl Pts',(0.205446825439215,-0.0126482899732578,
-0.226307022074615));
#25881=CARTESIAN_POINT('Ctrl Pts',(0.188370890182274,-0.0829746442192793,
-0.229959877021426));
#25882=CARTESIAN_POINT('Ctrl Pts',(0.145828951483188,-0.130510033480858,
-0.233612731968237));
#25883=CARTESIAN_POINT('Ctrl Pts',(0.103287012784103,-0.178045422742437,
-0.237265586915048));
#25884=CARTESIAN_POINT('Ctrl Pts',(0.0352790706428725,-0.202789847019573,
-0.24091844186186));
#25885=CARTESIAN_POINT('Ctrl Pts',(-0.0278631709630815,-0.193707423330989,
-0.244571296808671));
#25886=CARTESIAN_POINT('Ctrl Pts',(-0.091005412569035,-0.184624999642405,
-0.248224151755482));
#25887=CARTESIAN_POINT('Ctrl Pts',(-0.149281953639712,-0.141715727988102,
-0.251877006702293));
#25888=CARTESIAN_POINT('Ctrl Pts',(-0.176701220539749,-0.0841168822291211,
-0.255529861649104));
#25889=CARTESIAN_POINT('Ctrl Pts',(-0.18908613325676,-0.0581002611456236,
-0.257179806917484));
#25890=CARTESIAN_POINT('Ctrl Pts',(-0.195175523455146,-0.02908666294569,
-0.258829752185864));
#25891=CARTESIAN_POINT('Ctrl Pts',(-0.195110707760101,-4.72585694041849E-5,
-0.260479697454244));
#25892=CARTESIAN_POINT('Ctrl Pts',(-0.195100849729129,-1.92665112341343E-5,
-0.27065363587909));
#25893=CARTESIAN_POINT('Ctrl Pts',(-0.195130389340867,-0.0308561348349446,
-0.268901806567126));
#25894=CARTESIAN_POINT('Ctrl Pts',(-0.188229846664525,-0.0616807923984399,
-0.267149977255162));
#25895=CARTESIAN_POINT('Ctrl Pts',(-0.174327468766743,-0.0889330908388636,
-0.265398147943198));
#25896=CARTESIAN_POINT('Ctrl Pts',(-0.145338702835303,-0.145758657399616,
-0.261745292996387));
#25897=CARTESIAN_POINT('Ctrl Pts',(-0.0859065363182925,-0.187051901879128,
-0.258092438049576));
#25898=CARTESIAN_POINT('Ctrl Pts',(-0.022538802750656,-0.194398503605164,
-0.254439583102765));
#25899=CARTESIAN_POINT('Ctrl Pts',(0.0408289308169802,-0.201745105331199,
-0.250786728155954));
#25900=CARTESIAN_POINT('Ctrl Pts',(0.108132231435242,-0.175145064303758,
-0.247133873209142));
#25901=CARTESIAN_POINT('Ctrl Pts',(0.149354112356093,-0.126460722080181,
-0.243481018262331));
#25902=CARTESIAN_POINT('Ctrl Pts',(0.190575993276944,-0.077776379856603,
-0.23982816331552));
#25903=CARTESIAN_POINT('Ctrl Pts',(0.205716454500384,-0.00700773643688812,
-0.236175308368709));
#25904=CARTESIAN_POINT('Ctrl Pts',(0.188022556237584,0.0542814807221939,
-0.232522453421898));
#25905=CARTESIAN_POINT('Ctrl Pts',(0.170328657974784,0.115570697881275,
-0.228869598475086));
#25906=CARTESIAN_POINT('Ctrl Pts',(0.119800400225746,0.167380488779724,
-0.225216743528275));
#25907=CARTESIAN_POINT('Ctrl Pts',(0.0589736618385814,0.186603908499629,
-0.221563888581464));
#25908=CARTESIAN_POINT('Ctrl Pts',(-0.00185307654858394,0.205827328219534,
-0.217911033634653));
#25909=CARTESIAN_POINT('Ctrl Pts',(-0.072978295573876,0.192464376760895,
-0.214258178687842));
#25910=CARTESIAN_POINT('Ctrl Pts',(-0.122680009238483,0.152474774305509,
-0.21060532374103));
#25911=CARTESIAN_POINT('Ctrl Pts',(-0.167815111124156,0.116159431269827,
-0.207288094453717));
#25912=CARTESIAN_POINT('Ctrl Pts',(-0.195282649515434,0.0578855880163676,
-0.203970865166403));
#25913=CARTESIAN_POINT('Ctrl Pts',(-0.195637235488324,-9.58052375767378E-5,
-0.20065363587909));
#25914=CARTESIAN_POINT('Origin',(0.,0.,-0.19));
#25915=CARTESIAN_POINT('',(-0.195243803960011,0.00014500399526908,-0.120479697454244));
#25916=CARTESIAN_POINT('',(-0.19528814483522,0.000156602802769957,-0.13065363587909));
#25917=CARTESIAN_POINT('',(-0.1954,-2.39295984553393E-17,-0.19));
#25918=CARTESIAN_POINT('Ctrl Pts',(-0.195243803960011,0.00014500399526908,
-0.120479697454244));
#25919=CARTESIAN_POINT('Ctrl Pts',(-0.195392189818952,0.0209208269505307,
-0.121662159490796));
#25920=CARTESIAN_POINT('Ctrl Pts',(-0.192328368303915,0.0416539845471214,
-0.122844621527349));
#25921=CARTESIAN_POINT('Ctrl Pts',(-0.185863548863049,0.0612660467409409,
-0.124027083563902));
#25922=CARTESIAN_POINT('Ctrl Pts',(-0.165892465695211,0.121851516876383,
-0.127679938510713));
#25923=CARTESIAN_POINT('Ctrl Pts',(-0.113465247009462,0.171738237669897,
-0.131332793457524));
#25924=CARTESIAN_POINT('Ctrl Pts',(-0.0519631608745109,0.18867645654452,
-0.134985648404335));
#25925=CARTESIAN_POINT('Ctrl Pts',(0.00953892526044009,0.205614675419143,
-0.138638503351147));
#25926=CARTESIAN_POINT('Ctrl Pts',(0.0801158788445938,0.189604392374876,
-0.142291358297958));
#25927=CARTESIAN_POINT('Ctrl Pts',(0.128289431003563,0.147786308936136,
-0.145944213244769));
#25928=CARTESIAN_POINT('Ctrl Pts',(0.176462983162532,0.105968225497396,
-0.14959706819158));
#25929=CARTESIAN_POINT('Ctrl Pts',(0.202233133896316,0.0383423416641833,
-0.153249923138391));
#25930=CARTESIAN_POINT('Ctrl Pts',(0.194106710935588,-0.0249300405017104,
-0.156902778085202));
#25931=CARTESIAN_POINT('Ctrl Pts',(0.18598028797486,-0.0882024226676044,
-0.160555633032014));
#25932=CARTESIAN_POINT('Ctrl Pts',(0.143957291319619,-0.147121303166179,
-0.164208487978825));
#25933=CARTESIAN_POINT('Ctrl Pts',(0.086779895216793,-0.175408670583934,
-0.167861342925636));
#25934=CARTESIAN_POINT('Ctrl Pts',(0.0296024991139669,-0.20369603800169,
-0.171514197872447));
#25935=CARTESIAN_POINT('Ctrl Pts',(-0.0427292964364452,-0.201351892338625,
-0.175167052819258));
#25936=CARTESIAN_POINT('Ctrl Pts',(-0.0979551963305346,-0.169421743264796,
-0.178819907766069));
#25937=CARTESIAN_POINT('Ctrl Pts',(-0.153181096224624,-0.137491594190968,
-0.182472762712881));
#25938=CARTESIAN_POINT('Ctrl Pts',(-0.191301100462392,-0.0759754417063763,
-0.186125617659692));
#25939=CARTESIAN_POINT('Ctrl Pts',(-0.19531363165335,-0.0123096540548478,
-0.189778472606503));
#25940=CARTESIAN_POINT('Ctrl Pts',(-0.195570388501934,-0.00823575999095568,
-0.190012214222417));
#25941=CARTESIAN_POINT('Ctrl Pts',(-0.195687490258609,-0.00415306411707918,
-0.19024595583833));
#25942=CARTESIAN_POINT('Ctrl Pts',(-0.195668453670677,-6.92573205455238E-5,
-0.190479697454244));
#25943=CARTESIAN_POINT('Ctrl Pts',(-0.195637235488324,-9.58052375767378E-5,
-0.20065363587909));
#25944=CARTESIAN_POINT('Ctrl Pts',(-0.195673111257133,-0.00596215985583099,
-0.200318010219592));
#25945=CARTESIAN_POINT('Ctrl Pts',(-0.195431440278219,-0.0118255207556224,
-0.199982384560095));
#25946=CARTESIAN_POINT('Ctrl Pts',(-0.194902439849197,-0.0176628423614353,
-0.199646758900597));
#25947=CARTESIAN_POINT('Ctrl Pts',(-0.189144948491384,-0.0811946031208615,
-0.195993903953786));
#25948=CARTESIAN_POINT('Ctrl Pts',(-0.149351757471835,-0.14164187118758,
-0.192341049006975));
#25949=CARTESIAN_POINT('Ctrl Pts',(-0.0932707556744568,-0.172045046060018,
-0.188688194060163));
#25950=CARTESIAN_POINT('Ctrl Pts',(-0.0371897538770789,-0.202448220932456,
-0.185035339113352));
#25951=CARTESIAN_POINT('Ctrl Pts',(0.0351790586981286,-0.202807302610614,
-0.181382484166541));
#25952=CARTESIAN_POINT('Ctrl Pts',(0.0915589780120191,-0.17296210786544,
-0.17772962921973));
#25953=CARTESIAN_POINT('Ctrl Pts',(0.14793889732591,-0.143116913120265,
-0.174076774272919));
#25954=CARTESIAN_POINT('Ctrl Pts',(0.188329923378484,-0.0830674419517585,
-0.170423919326108));
#25955=CARTESIAN_POINT('Ctrl Pts',(0.194717565566022,-0.0195959536108856,
-0.166771064379296));
#25956=CARTESIAN_POINT('Ctrl Pts',(0.20110520775356,0.043875534729987,-0.163118209432485));
#25957=CARTESIAN_POINT('Ctrl Pts',(0.173489466076062,0.110769040243225,
-0.159465354485674));
#25958=CARTESIAN_POINT('Ctrl Pts',(0.124186989019549,0.151249888653556,
-0.155812499538863));
#25959=CARTESIAN_POINT('Ctrl Pts',(0.0748845119630359,0.191730737063888,
-0.152159644592052));
#25960=CARTESIAN_POINT('Ctrl Pts',(0.00389529952750602,0.205798928371311,
-0.148506789645241));
#25961=CARTESIAN_POINT('Ctrl Pts',(-0.0571191521156268,0.187179977369007,
-0.144853934698429));
#25962=CARTESIAN_POINT('Ctrl Pts',(-0.118133603758759,0.168561026366703,
-0.141201079751618));
#25963=CARTESIAN_POINT('Ctrl Pts',(-0.169173294609495,0.117254933054672,
-0.137548224804807));
#25964=CARTESIAN_POINT('Ctrl Pts',(-0.187474573932762,0.0561444172355426,
-0.133895369857996));
#25965=CARTESIAN_POINT('Ctrl Pts',(-0.192888410498366,0.0380668643366071,
-0.132814791865027));
#25966=CARTESIAN_POINT('Ctrl Pts',(-0.195437376622097,0.0191313467738501,
-0.131734213872058));
#25967=CARTESIAN_POINT('Ctrl Pts',(-0.19528814483522,0.000156602802769957,
-0.13065363587909));
#25968=CARTESIAN_POINT('Origin',(0.,0.,-0.19));
#25969=CARTESIAN_POINT('',(-0.195345140381879,-0.000154736422984442,-0.0504796974542436));
#25970=CARTESIAN_POINT('',(-0.195260766042512,-0.000146819403851512,-0.0606536358790897));
#25971=CARTESIAN_POINT('',(-0.1954,-2.39295984553393E-17,-0.19));
#25972=CARTESIAN_POINT('Ctrl Pts',(-0.195345140381879,-0.000154736422984442,
-0.0504796974542436));
#25973=CARTESIAN_POINT('Ctrl Pts',(-0.194969681403942,0.0454695115731484,
-0.0530783631432626));
#25974=CARTESIAN_POINT('Ctrl Pts',(-0.178930944341532,0.0913218023900443,
-0.0556770288322816));
#25975=CARTESIAN_POINT('Ctrl Pts',(-0.149690022397842,0.126037510600571,
-0.0582756945213006));
#25976=CARTESIAN_POINT('Ctrl Pts',(-0.108587064513464,0.174836187169372,
-0.0619285494681118));
#25977=CARTESIAN_POINT('Ctrl Pts',(-0.0413979655074079,0.201630137392092,
-0.065581404414923));
#25978=CARTESIAN_POINT('Ctrl Pts',(0.0219807109386058,0.194462607355388,
-0.0692342593617342));
#25979=CARTESIAN_POINT('Ctrl Pts',(0.0853593873846187,0.187295077318685,
-0.0728871143085453));
#25980=CARTESIAN_POINT('Ctrl Pts',(0.14492764127059,0.146166067022559,-0.0765399692553564));
#25981=CARTESIAN_POINT('Ctrl Pts',(0.174081505004941,0.089422596913196,
-0.0801928242021676));
#25982=CARTESIAN_POINT('Ctrl Pts',(0.203235368739293,0.0326791268038316,
-0.0838456791489788));
#25983=CARTESIAN_POINT('Ctrl Pts',(0.201974842322025,-0.0396788031187714,
-0.08749853409579));
#25984=CARTESIAN_POINT('Ctrl Pts',(0.17088111660692,-0.0953810986953389,
-0.0911513890426013));
#25985=CARTESIAN_POINT('Ctrl Pts',(0.139787390891815,-0.151083394271906,
-0.0948042439894125));
#25986=CARTESIAN_POINT('Ctrl Pts',(0.0788604658788755,-0.190130055502438,
-0.0984570989362236));
#25987=CARTESIAN_POINT('Ctrl Pts',(0.0152639920062928,-0.195105243720415,
-0.102109953883035));
#25988=CARTESIAN_POINT('Ctrl Pts',(-0.04833248186629,-0.200080431938393,
-0.105762808829846));
#25989=CARTESIAN_POINT('Ctrl Pts',(-0.114598504598516,-0.170984147143816,
-0.109415663776657));
#25990=CARTESIAN_POINT('Ctrl Pts',(-0.153974042139665,-0.120793895007844,
-0.113068518723468));
#25991=CARTESIAN_POINT('Ctrl Pts',(-0.180603363641792,-0.0868506794008215,
-0.115538911633727));
#25992=CARTESIAN_POINT('Ctrl Pts',(-0.194933797073887,-0.0432597262598245,
-0.118009304543985));
#25993=CARTESIAN_POINT('Ctrl Pts',(-0.195243803960011,0.00014500399526908,
-0.120479697454244));
#25994=CARTESIAN_POINT('Ctrl Pts',(-0.19528814483522,0.000156602802769957,
-0.13065363587909));
#25995=CARTESIAN_POINT('Ctrl Pts',(-0.194932903946858,-0.0450120911179513,
-0.128081358925247));
#25996=CARTESIAN_POINT('Ctrl Pts',(-0.179288031569788,-0.0904030657414807,
-0.125509081971405));
#25997=CARTESIAN_POINT('Ctrl Pts',(-0.150601799725115,-0.124972231807972,
-0.122936805017562));
#25998=CARTESIAN_POINT('Ctrl Pts',(-0.109864878398407,-0.17406342670613,
-0.119283950070751));
#25999=CARTESIAN_POINT('Ctrl Pts',(-0.042828167949195,-0.20133087817622,
-0.11563109512394));
#26000=CARTESIAN_POINT('Ctrl Pts',(0.0206090388069535,-0.194613033032659,
-0.111978240177129));
#26001=CARTESIAN_POINT('Ctrl Pts',(0.0840462455631022,-0.187895187889097,
-0.108325385230318));
#26002=CARTESIAN_POINT('Ctrl Pts',(0.143883948626187,-0.147192046131885,
-0.104672530283506));
#26003=CARTESIAN_POINT('Ctrl Pts',(0.173435748689723,-0.0906576908474678,
-0.101019675336695));
#26004=CARTESIAN_POINT('Ctrl Pts',(0.202987548753259,-0.03412333556305,
-0.097366820389884));
#26005=CARTESIAN_POINT('Ctrl Pts',(0.202253445817245,0.0382422332485734,
-0.0937139654430728));
#26006=CARTESIAN_POINT('Ctrl Pts',(0.171558198859466,0.0941644594147348,
-0.0900611104962616));
#26007=CARTESIAN_POINT('Ctrl Pts',(0.140862951901687,0.150086685580896,
-0.0864082555494504));
#26008=CARTESIAN_POINT('Ctrl Pts',(0.0802065609221434,0.189565569101596,
-0.0827554006026392));
#26009=CARTESIAN_POINT('Ctrl Pts',(0.0166470195008158,0.194992084644279,
-0.079102545655828));
#26010=CARTESIAN_POINT('Ctrl Pts',(-0.0469125219205106,0.200418600186961,
-0.0754496907090168));
#26011=CARTESIAN_POINT('Ctrl Pts',(-0.113375213783621,0.171792747751628,
-0.0717968357622057));
#26012=CARTESIAN_POINT('Ctrl Pts',(-0.153108187162892,0.121884280074465,
-0.0681439808153946));
#26013=CARTESIAN_POINT('Ctrl Pts',(-0.180266275862396,0.0877710870069687,
-0.0656471991699597));
#26014=CARTESIAN_POINT('Ctrl Pts',(-0.194936428770792,0.0437148063320393,
-0.0631504175245247));
#26015=CARTESIAN_POINT('Ctrl Pts',(-0.195260766042512,-0.000146819403851512,
-0.0606536358790897));
#26016=CARTESIAN_POINT('Origin',(0.,0.,-0.482472289227037));
#26017=CARTESIAN_POINT('',(-0.155506328487213,-0.000123179378687057,-0.0274722892270369));
#26018=CARTESIAN_POINT('',(-0.15555,-6.69085778714157E-17,-0.0253999999999999));
#26019=CARTESIAN_POINT('',(-0.15555,-6.69085778714157E-17,-0.482472289227037));
#26020=CARTESIAN_POINT('',(-0.152866807250001,-0.0287670252405615,-0.0254));
#26021=CARTESIAN_POINT('Ctrl Pts',(-0.155506328487213,-0.000123179378687057,
-0.0274722892270369));
#26022=CARTESIAN_POINT('Ctrl Pts',(-0.155585777160968,-0.00977745909336126,
-0.0267815261513579));
#26023=CARTESIAN_POINT('Ctrl Pts',(-0.154784206338799,-0.0194189119802211,
-0.026090763075679));
#26024=CARTESIAN_POINT('Ctrl Pts',(-0.153064819257014,-0.0288776210951403,
-0.0254));
#26025=CARTESIAN_POINT('Origin',(0.,0.,-0.0254));
#26026=CARTESIAN_POINT('Origin',(0.,0.,-0.482472289227037));
#26027=CARTESIAN_POINT('',(-0.155425658679527,0.000115431788456025,-0.097472289227037));
#26028=CARTESIAN_POINT('',(-0.15543916150416,-0.000116876961459109,-0.0836610441062964));
#26029=CARTESIAN_POINT('',(-0.15555,-6.69085778714157E-17,-0.482472289227037));
#26030=CARTESIAN_POINT('Ctrl Pts',(-0.155425658679527,0.000115431788456041,
-0.097472289227037));
#26031=CARTESIAN_POINT('Ctrl Pts',(-0.155178874794489,-0.0344373102339589,
-0.0950018963167785));
#26032=CARTESIAN_POINT('Ctrl Pts',(-0.126902704468458,-0.120449029386036,
-0.0888786484597088));
#26033=CARTESIAN_POINT('Ctrl Pts',(0.0142761631611888,-0.182438271687888,
-0.0791025456558283));
#26034=CARTESIAN_POINT('Ctrl Pts',(0.159780510946698,-0.0891878906068867,
-0.0681439808153946));
#26035=CARTESIAN_POINT('Ctrl Pts',(0.162790872526117,0.083615732721579,
-0.0571854159749611));
#26036=CARTESIAN_POINT('Ctrl Pts',(0.0205312733659909,0.181839134229702,
-0.0462268511345275));
#26037=CARTESIAN_POINT('Ctrl Pts',(-0.124492415332785,0.124005980435514,
-0.0363224755518862));
#26038=CARTESIAN_POINT('Ctrl Pts',(-0.155207440851501,0.0361964305281632,
-0.0300709549160559));
#26039=CARTESIAN_POINT('Ctrl Pts',(-0.155506328487213,-0.000123179378687057,
-0.0274722892270369));
#26040=CARTESIAN_POINT('',(-0.0768992790589743,0.135212068175182,-0.0253999999999999));
#26041=CARTESIAN_POINT('Origin',(0.,0.,-0.0254));
#26042=CARTESIAN_POINT('Ctrl Pts',(-0.15543916150416,-0.000116876961459117,
-0.0836610441062964));
#26043=CARTESIAN_POINT('Ctrl Pts',(-0.155558710827905,-0.0162840836081317,
-0.0825049708049201));
#26044=CARTESIAN_POINT('Ctrl Pts',(-0.145871418380864,-0.0833967626835857,
-0.0776960425567327));
#26045=CARTESIAN_POINT('Ctrl Pts',(-0.0498103614642923,-0.176085032876655,
-0.069234259361734));
#26046=CARTESIAN_POINT('Ctrl Pts',(0.118915079055016,-0.139024368591976,
-0.0582756945213005));
#26047=CARTESIAN_POINT('Ctrl Pts',(0.18178171708891,0.0219900978007506,
-0.0473171296808669));
#26048=CARTESIAN_POINT('Ctrl Pts',(0.0820716217526228,0.163506105608369,
-0.0363585648404334));
#26049=CARTESIAN_POINT('Ctrl Pts',(-0.0325660146575313,0.160425764828242,
-0.0290528549468111));
#26050=CARTESIAN_POINT('Ctrl Pts',(-0.0768992790589753,0.135212068175181,
-0.0253999999999999));
#26051=CARTESIAN_POINT('Origin',(0.,0.,-0.482472289227037));
#26052=CARTESIAN_POINT('',(-0.155763705058719,-5.51329386419761E-5,-0.167472289227037));
#26053=CARTESIAN_POINT('',(-0.155460956648508,0.00012466512779525,-0.153661044106296));
#26054=CARTESIAN_POINT('',(-0.15555,-6.69085778714157E-17,-0.482472289227037));
#26055=CARTESIAN_POINT('Ctrl Pts',(-0.155763705058719,-5.51329386419977E-5,
-0.167472289227037));
#26056=CARTESIAN_POINT('Ctrl Pts',(-0.155778859312828,-0.00330608558552471,
-0.167238547611123));
#26057=CARTESIAN_POINT('Ctrl Pts',(-0.154228821523255,-0.0573474003148411,
-0.163351951048399));
#26058=CARTESIAN_POINT('Ctrl Pts',(-0.0915954598697826,-0.158421980529086,
-0.155812499538863));
#26059=CARTESIAN_POINT('Ctrl Pts',(0.081145749923459,-0.16402021785595,
-0.144853934698429));
#26060=CARTESIAN_POINT('Ctrl Pts',(0.181504150072734,-0.0233114379958674,
-0.133895369857996));
#26061=CARTESIAN_POINT('Ctrl Pts',(0.119960440554205,0.138191216511648,
-0.122936805017562));
#26062=CARTESIAN_POINT('Ctrl Pts',(-0.0485898940929054,0.176426623792137,
-0.111978240177129));
#26063=CARTESIAN_POINT('Ctrl Pts',(-0.145570304009841,0.0841456530817482,
-0.103490068246954));
#26064=CARTESIAN_POINT('Ctrl Pts',(-0.155543782632231,0.0166542202259733,
-0.0986547512635898));
#26065=CARTESIAN_POINT('Ctrl Pts',(-0.155425658679527,0.000115431788456041,
-0.097472289227037));
#26066=CARTESIAN_POINT('Ctrl Pts',(-0.155460956648508,0.000124665127795244,
-0.153661044106296));
#26067=CARTESIAN_POINT('Ctrl Pts',(-0.155178163812353,-0.0358322966908755,
-0.151088767152454));
#26068=CARTESIAN_POINT('Ctrl Pts',(-0.125037812369975,-0.123279473918762,
-0.1448636352518));
#26069=CARTESIAN_POINT('Ctrl Pts',(0.0192714369799267,-0.181977841230724,
-0.134985648404336));
#26070=CARTESIAN_POINT('Ctrl Pts',(0.162174528762878,-0.0847714896391007,
-0.124027083563902));
#26071=CARTESIAN_POINT('Ctrl Pts',(0.160421360210723,0.0880503767168045,
-0.113068518723468));
#26072=CARTESIAN_POINT('Ctrl Pts',(0.0155630958780523,0.182332981603879,
-0.102109953883035));
#26073=CARTESIAN_POINT('Ctrl Pts',(-0.126416989269986,0.12118136627998,
-0.0923074623439774));
#26074=CARTESIAN_POINT('Ctrl Pts',(-0.155180969781457,0.0347995809874546,
-0.0861578257517313));
#26075=CARTESIAN_POINT('Ctrl Pts',(-0.15543916150416,-0.000116876961459117,
-0.0836610441062964));
#26076=CARTESIAN_POINT('Origin',(0.,0.,-0.482472289227037));
#26077=CARTESIAN_POINT('',(-0.15531970620309,-3.76206267698384E-5,-0.237472289227037));
#26078=CARTESIAN_POINT('',(-0.155738853532286,-7.62666566272302E-5,-0.223661044106296));
#26079=CARTESIAN_POINT('',(-0.15555,-6.69085778714157E-17,-0.482472289227037));
#26080=CARTESIAN_POINT('Ctrl Pts',(-0.15531970620309,-3.76206267698534E-5,
-0.237472289227037));
#26081=CARTESIAN_POINT('Ctrl Pts',(-0.155371303344155,-0.0231547104462748,
-0.235822343958657));
#26082=CARTESIAN_POINT('Ctrl Pts',(-0.139791750558325,-0.0973852770443118,
-0.230519543743466));
#26083=CARTESIAN_POINT('Ctrl Pts',(-0.0260541246753813,-0.181130787616187,
-0.221563888581464));
#26084=CARTESIAN_POINT('Ctrl Pts',(0.136360953114818,-0.122036695554133,
-0.21060532374103));
#26085=CARTESIAN_POINT('Ctrl Pts',(0.177141327667794,0.0459151632427247,
-0.199646758900597));
#26086=CARTESIAN_POINT('Ctrl Pts',(0.0599105989065099,0.172910257764587,
-0.188688194060163));
#26087=CARTESIAN_POINT('Ctrl Pts',(-0.107120389660789,0.146249553923857,
-0.177963370835644));
#26088=CARTESIAN_POINT('Ctrl Pts',(-0.155542032456515,0.0474989814180707,
-0.170891402557935));
#26089=CARTESIAN_POINT('Ctrl Pts',(-0.155763705058719,-5.51329386419977E-5,
-0.167472289227037));
#26090=CARTESIAN_POINT('Ctrl Pts',(-0.155738853532286,-7.62666566272467E-5,
-0.223661044106297));
#26091=CARTESIAN_POINT('Ctrl Pts',(-0.155767412774038,-0.00474623319127167,
-0.223325418446799));
#26092=CARTESIAN_POINT('Ctrl Pts',(-0.153481170317431,-0.0602144763693775,
-0.21933693784049));
#26093=CARTESIAN_POINT('Ctrl Pts',(-0.0872151228846113,-0.160874951949878,
-0.21169560228737));
#26094=CARTESIAN_POINT('Ctrl Pts',(0.0856144901564349,-0.161732502948406,
-0.200737037446937));
#26095=CARTESIAN_POINT('Ctrl Pts',(0.182075453858757,-0.01832367121461,
-0.189778472606503));
#26096=CARTESIAN_POINT('Ctrl Pts',(0.116124144473882,0.141429933431004,
-0.178819907766069));
#26097=CARTESIAN_POINT('Ctrl Pts',(-0.0534107377320515,0.175027279764724,
-0.167861342925636));
#26098=CARTESIAN_POINT('Ctrl Pts',(-0.146691230408257,0.081259908104232,
-0.159475055039045));
#26099=CARTESIAN_POINT('Ctrl Pts',(-0.155579754010068,0.0152296877721218,
-0.154741622099265));
#26100=CARTESIAN_POINT('Ctrl Pts',(-0.155460956648508,0.000124665127795244,
-0.153661044106296));
#26101=CARTESIAN_POINT('Origin',(0.,0.,-0.482472289227037));
#26102=CARTESIAN_POINT('',(-0.155653088469525,0.000125523659554109,-0.307472289227037));
#26103=CARTESIAN_POINT('',(-0.15531185862521,-1.53372867060936E-5,-0.293661044106296));
#26104=CARTESIAN_POINT('',(-0.15555,-6.69085778714157E-17,-0.482472289227037));
#26105=CARTESIAN_POINT('Ctrl Pts',(-0.155653088469525,0.000125523659554115,
-0.307472289227037));
#26106=CARTESIAN_POINT('Ctrl Pts',(-0.155297443306996,-0.0425972855119035,
-0.304406140306191));
#26107=CARTESIAN_POINT('Ctrl Pts',(-0.115130098271041,-0.136833824827096,
-0.297687136438534));
#26108=CARTESIAN_POINT('Ctrl Pts',(0.0432320574545622,-0.177806863527647,
-0.287315277624065));
#26109=CARTESIAN_POINT('Ctrl Pts',(0.171983496481539,-0.0625236655119731,
-0.276356712783632));
#26110=CARTESIAN_POINT('Ctrl Pts',(0.147327574909702,0.10854710720198,-0.265398147943198));
#26111=CARTESIAN_POINT('Ctrl Pts',(-0.00874691461069841,0.182784808841176,
-0.254439583102765));
#26112=CARTESIAN_POINT('Ctrl Pts',(-0.134694247358807,0.107352187029585,
-0.245130963530711));
#26113=CARTESIAN_POINT('Ctrl Pts',(-0.155257071147734,0.0280247907901394,
-0.239475198905468));
#26114=CARTESIAN_POINT('Ctrl Pts',(-0.15531970620309,-3.76206267698534E-5,
-0.237472289227037));
#26115=CARTESIAN_POINT('Ctrl Pts',(-0.15531185862521,-1.5337286706104E-5,
-0.293661044106296));
#26116=CARTESIAN_POINT('Ctrl Pts',(-0.155335373909784,-0.0245633151155352,
-0.291909214794333));
#26117=CARTESIAN_POINT('Ctrl Pts',(-0.138387811535161,-0.100267912744467,
-0.286504530535558));
#26118=CARTESIAN_POINT('Ctrl Pts',(-0.0210751700234872,-0.18177629230341,
-0.277446991329971));
#26119=CARTESIAN_POINT('Ctrl Pts',(0.139657098315878,-0.118250656963312,
-0.266488426489538));
#26120=CARTESIAN_POINT('Ctrl Pts',(0.175815216176257,0.0507574671503514,
-0.255529861649104));
#26121=CARTESIAN_POINT('Ctrl Pts',(0.0551447377802041,0.174488474943397,
-0.244571296808671));
#26122=CARTESIAN_POINT('Ctrl Pts',(-0.109512695395071,0.143552763011982,
-0.233948357627735));
#26123=CARTESIAN_POINT('Ctrl Pts',(-0.155456582047726,0.0460803644623646,
-0.22697827339361));
#26124=CARTESIAN_POINT('Ctrl Pts',(-0.155738853532286,-7.62666566272467E-5,
-0.223661044106297));
#26125=CARTESIAN_POINT('Origin',(2.59090492670967E-17,0.,-0.0254));
#26126=CARTESIAN_POINT('',(0.122919639333555,-0.151894444487311,-0.0254));
#26127=CARTESIAN_POINT('Ctrl Pts',(-0.153064819257014,-0.0288776210951403,
-0.0254));
#26128=CARTESIAN_POINT('Ctrl Pts',(-0.152777592917439,-0.0340072377393832,
-0.0254));
#26129=CARTESIAN_POINT('Ctrl Pts',(-0.152223882228274,-0.0391080712845753,
-0.0254));
#26130=CARTESIAN_POINT('Ctrl Pts',(-0.151399448027242,-0.0441601340310789,
-0.0254));
#26131=CARTESIAN_POINT('Ctrl Pts',(-0.150330370732434,-0.0507113488733025,
-0.0254));
#26132=CARTESIAN_POINT('Ctrl Pts',(-0.14880642391072,-0.0571806323888862,
-0.0253999999999999));
#26133=CARTESIAN_POINT('Ctrl Pts',(-0.146862321130527,-0.063540143599143,
-0.0254));
#26134=CARTESIAN_POINT('Ctrl Pts',(-0.145388672016564,-0.0683607159246997,
-0.0254));
#26135=CARTESIAN_POINT('Ctrl Pts',(-0.143671994693297,-0.0731203555579338,
-0.0253999999999997));
#26136=CARTESIAN_POINT('Ctrl Pts',(-0.141735119284282,-0.0777852836788175,
-0.0253999999999998));
#26137=CARTESIAN_POINT('Ctrl Pts',(-0.138078365687791,-0.0865925061795565,
-0.0253999999999999));
#26138=CARTESIAN_POINT('Ctrl Pts',(-0.133634254588353,-0.0950791659576873,
-0.0253999999999999));
#26139=CARTESIAN_POINT('Ctrl Pts',(-0.128494059306883,-0.103165599018055,
-0.0253999999999999));
#26140=CARTESIAN_POINT('Ctrl Pts',(-0.126025864689144,-0.10704850413418,
-0.0253999999999999));
#26141=CARTESIAN_POINT('Ctrl Pts',(-0.123395149747612,-0.110840498855916,
-0.0253999999999999));
#26142=CARTESIAN_POINT('Ctrl Pts',(-0.120624606677722,-0.114514842153386,
-0.0253999999999999));
#26143=CARTESIAN_POINT('Ctrl Pts',(-0.113588026278536,-0.123846879726758,
-0.0253999999999999));
#26144=CARTESIAN_POINT('Ctrl Pts',(-0.105637653785234,-0.132447744046583,
-0.0253999999999999));
#26145=CARTESIAN_POINT('Ctrl Pts',(-0.0969241262231594,-0.140179311463173,
-0.0253999999999999));
#26146=CARTESIAN_POINT('Ctrl Pts',(-0.09294324074945,-0.14371157600224,
-0.0253999999999999));
#26147=CARTESIAN_POINT('Ctrl Pts',(-0.0888023607437844,-0.147062196487114,
-0.0254));
#26148=CARTESIAN_POINT('Ctrl Pts',(-0.0845127230821876,-0.150216270470207,
-0.0254));
#26149=CARTESIAN_POINT('Ctrl Pts',(-0.0807618339747387,-0.152974214772399,
-0.0254));
#26150=CARTESIAN_POINT('Ctrl Pts',(-0.0768933726595271,-0.155583707402879,
-0.0253999999999999));
#26151=CARTESIAN_POINT('Ctrl Pts',(-0.0729386575525788,-0.158019936339133,
-0.0253999999999999));
#26152=CARTESIAN_POINT('Ctrl Pts',(-0.0664307842915506,-0.162028991030365,
-0.0253999999999999));
#26153=CARTESIAN_POINT('Ctrl Pts',(-0.0596792629904233,-0.165577918385484,
-0.0253999999999999));
#26154=CARTESIAN_POINT('Ctrl Pts',(-0.0527219813591869,-0.168628838889641,
-0.0253999999999999));
#26155=CARTESIAN_POINT('Ctrl Pts',(-0.0455901588913395,-0.17175629937672,
-0.0254));
#26156=CARTESIAN_POINT('Ctrl Pts',(-0.0382420298855482,-0.174360754422375,
-0.0254));
#26157=CARTESIAN_POINT('Ctrl Pts',(-0.0307291264526019,-0.176457918562462,
-0.0254));
#26158=CARTESIAN_POINT('Ctrl Pts',(-0.0265471472130843,-0.177625283080584,
-0.0254));
#26159=CARTESIAN_POINT('Ctrl Pts',(-0.0223140014545879,-0.178635304140707,
-0.0253999999999999));
#26160=CARTESIAN_POINT('Ctrl Pts',(-0.0180379599774122,-0.179489460836271,
-0.0253999999999999));
#26161=CARTESIAN_POINT('Ctrl Pts',(-0.0145498200543281,-0.180186230988354,
-0.0253999999999999));
#26162=CARTESIAN_POINT('Ctrl Pts',(-0.0110380948897776,-0.180778117133158,
-0.0254000000000001));
#26163=CARTESIAN_POINT('Ctrl Pts',(-0.0075153478077699,-0.181265734494698,
-0.0254000000000001));
#26164=CARTESIAN_POINT('Ctrl Pts',(0.00372069158298919,-0.182821022954056,
-0.0254));
#26165=CARTESIAN_POINT('Ctrl Pts',(0.0150906888787215,-0.183322996861398,
-0.0254));
#26166=CARTESIAN_POINT('Ctrl Pts',(0.0264435674523557,-0.182817859387596,
-0.0254));
#26167=CARTESIAN_POINT('Ctrl Pts',(0.0340855280180532,-0.182477836315033,
-0.0254000000000001));
#26168=CARTESIAN_POINT('Ctrl Pts',(0.0417202563974908,-0.181680756711447,
-0.0254));
#26169=CARTESIAN_POINT('Ctrl Pts',(0.0493042471779824,-0.180431503266826,
-0.0254));
#26170=CARTESIAN_POINT('Ctrl Pts',(0.0532122465331841,-0.17978776808869,
-0.0254));
#26171=CARTESIAN_POINT('Ctrl Pts',(0.0571088690032366,-0.179023120919283,
-0.0254));
#26172=CARTESIAN_POINT('Ctrl Pts',(0.0609702128695543,-0.178142282480996,
-0.0254));
#26173=CARTESIAN_POINT('Ctrl Pts',(0.0734785721675836,-0.175288912242277,
-0.0254000000000001));
#26174=CARTESIAN_POINT('Ctrl Pts',(0.0856546858321524,-0.171215349953341,
-0.0254));
#26175=CARTESIAN_POINT('Ctrl Pts',(0.0973011784066163,-0.165963075675207,
-0.0254));
#26176=CARTESIAN_POINT('Ctrl Pts',(0.106177882671306,-0.161959906035425,
-0.0254));
#26177=CARTESIAN_POINT('Ctrl Pts',(0.114747547478628,-0.157270963555419,
-0.0254));
#26178=CARTESIAN_POINT('Ctrl Pts',(0.122919639333555,-0.151894444487311,
-0.0254));
#26179=CARTESIAN_POINT('',(-0.1954,-2.39295984553393E-17,-0.0254));
#26180=CARTESIAN_POINT('Origin',(0.,0.,-0.0254));
#26181=CARTESIAN_POINT('',(0.195483386661889,0.00449643670064488,-0.0254));
#26182=CARTESIAN_POINT('Origin',(0.,0.,-0.0254));
#26183=CARTESIAN_POINT('Ctrl Pts',(0.1956174094926,0.00454472201517893,
-0.0254));
#26184=CARTESIAN_POINT('Ctrl Pts',(0.194884502242902,0.0108609228279264,
-0.0254));
#26185=CARTESIAN_POINT('Ctrl Pts',(0.193827694703694,0.0171246191869846,
-0.0254));
#26186=CARTESIAN_POINT('Ctrl Pts',(0.192436221146521,0.0233138906391813,
-0.0254));
#26187=CARTESIAN_POINT('Ctrl Pts',(0.190305921538478,0.0327894588098559,
-0.0254));
#26188=CARTESIAN_POINT('Ctrl Pts',(0.187391725008866,0.0420911964277299,
-0.0254000000000001));
#26189=CARTESIAN_POINT('Ctrl Pts',(0.183750788578834,0.0511458524301873,
-0.0254000000000001));
#26190=CARTESIAN_POINT('Ctrl Pts',(0.182256333478902,0.0548624174131394,
-0.0254000000000001));
#26191=CARTESIAN_POINT('Ctrl Pts',(0.180639878796232,0.0585352549444029,
-0.0254));
#26192=CARTESIAN_POINT('Ctrl Pts',(0.178909447829662,0.0621511985197291,
-0.0254));
#26193=CARTESIAN_POINT('Ctrl Pts',(0.175759243024173,0.0687339302480849,
-0.0254));
#26194=CARTESIAN_POINT('Ctrl Pts',(0.172228441682624,0.0751362936533435,
-0.0254));
#26195=CARTESIAN_POINT('Ctrl Pts',(0.168341962135569,0.081327087720111,
-0.0254000000000001));
#26196=CARTESIAN_POINT('Ctrl Pts',(0.165097336199203,0.0864954697359009,
-0.0254000000000001));
#26197=CARTESIAN_POINT('Ctrl Pts',(0.161604700724613,0.0915163594823662,
-0.0254000000000001));
#26198=CARTESIAN_POINT('Ctrl Pts',(0.157876721750264,0.0963691400874196,
-0.0254000000000002));
#26199=CARTESIAN_POINT('Ctrl Pts',(0.155393249616941,0.0996019226445926,
-0.0254000000000002));
#26200=CARTESIAN_POINT('Ctrl Pts',(0.152811199634149,0.102752305844702,
-0.0254));
#26201=CARTESIAN_POINT('Ctrl Pts',(0.15013686171718,0.105813287041844,-0.0254));
#26202=CARTESIAN_POINT('Ctrl Pts',(0.142106471379143,0.115004673692902,
-0.0254));
#26203=CARTESIAN_POINT('Ctrl Pts',(0.133241108450999,0.123399305600953,
-0.0254));
#26204=CARTESIAN_POINT('Ctrl Pts',(0.123649781692531,0.130835395348286,
-0.0254000000000001));
#26205=CARTESIAN_POINT('Ctrl Pts',(0.119112362619058,0.134353225185729,
-0.0254000000000001));
#26206=CARTESIAN_POINT('Ctrl Pts',(0.114412125674294,0.137655883629633,
-0.0253999999999999));
#26207=CARTESIAN_POINT('Ctrl Pts',(0.109559388770948,0.140722179479723,
-0.0253999999999999));
#26208=CARTESIAN_POINT('Ctrl Pts',(0.106359640552875,0.14274400239694,-0.0253999999999999));
#26209=CARTESIAN_POINT('Ctrl Pts',(0.103091731428373,0.144663720869763,
-0.0254));
#26210=CARTESIAN_POINT('Ctrl Pts',(0.0997741086716124,0.146466938326076,
-0.0254));
#26211=CARTESIAN_POINT('Ctrl Pts',(0.0929232199256937,0.150190581152171,
-0.0254));
#26212=CARTESIAN_POINT('Ctrl Pts',(0.0858475401072859,0.153427047025761,
-0.0254));
#26213=CARTESIAN_POINT('Ctrl Pts',(0.078575952192563,0.156129623366496,
-0.0254));
#26214=CARTESIAN_POINT('Ctrl Pts',(0.0721329233957311,0.158524255377166,
-0.0254));
#26215=CARTESIAN_POINT('Ctrl Pts',(0.0655359016892521,0.160499536766023,
-0.0254));
#26216=CARTESIAN_POINT('Ctrl Pts',(0.0588237208555869,0.162058462470114,
-0.0254));
#26217=CARTESIAN_POINT('Ctrl Pts',(0.0538349286583048,0.163217125590407,
-0.0254));
#26218=CARTESIAN_POINT('Ctrl Pts',(0.0487825015420083,0.164145657243952,
-0.0254));
#26219=CARTESIAN_POINT('Ctrl Pts',(0.0436829085690683,0.164843212472954,
-0.0254));
#26220=CARTESIAN_POINT('Ctrl Pts',(0.039963114449189,0.165352029912483,
-0.0254));
#26221=CARTESIAN_POINT('Ctrl Pts',(0.0362254315579577,0.165736782759396,
-0.0254));
#26222=CARTESIAN_POINT('Ctrl Pts',(0.0324835004058875,0.165997995639231,
-0.0254));
#26223=CARTESIAN_POINT('Ctrl Pts',(0.0228345603237951,0.1666715589208,-0.0254000000000001));
#26224=CARTESIAN_POINT('Ctrl Pts',(0.0131416919040143,0.166527582794073,
-0.0254));
#26225=CARTESIAN_POINT('Ctrl Pts',(0.00351603350894282,0.165574729310518,
-0.0254));
#26226=CARTESIAN_POINT('Ctrl Pts',(-0.00271730357169677,0.164957685082718,
-0.0253999999999999));
#26227=CARTESIAN_POINT('Ctrl Pts',(-0.00892239601177496,0.164000905828904,
-0.0254));
#26228=CARTESIAN_POINT('Ctrl Pts',(-0.0150663391055822,0.16270149682046,
-0.0254000000000001));
#26229=CARTESIAN_POINT('Ctrl Pts',(-0.0195365657371929,0.161756069321179,
-0.0254000000000001));
#26230=CARTESIAN_POINT('Ctrl Pts',(-0.0239783961275451,0.160627551616827,
-0.0253999999999999));
#26231=CARTESIAN_POINT('Ctrl Pts',(-0.0283517173245239,0.159322701788556,
-0.0254));
#26232=CARTESIAN_POINT('Ctrl Pts',(-0.0386808148966284,0.156240851499933,
-0.0254));
#26233=CARTESIAN_POINT('Ctrl Pts',(-0.0486583234698455,0.15217404561927,
-0.0254000000000001));
#26234=CARTESIAN_POINT('Ctrl Pts',(-0.0581163771297697,0.147117423395272,
-0.0254));
#26235=CARTESIAN_POINT('Ctrl Pts',(-0.0646475390281869,0.143625624808423,
-0.0254));
#26236=CARTESIAN_POINT('Ctrl Pts',(-0.0709305950931194,0.139660961676877,
-0.0254));
#26237=CARTESIAN_POINT('Ctrl Pts',(-0.0768992790589734,0.135212068175182,
-0.0254));
#26238=CARTESIAN_POINT('Ctrl Pts',(-0.0685825729128703,0.139614588036676,
-0.376074074893873));
#26239=CARTESIAN_POINT('Ctrl Pts',(-0.114359333295748,0.117127768780733,
-0.372421219947062));
#26240=CARTESIAN_POINT('Ctrl Pts',(-0.181359531123569,0.0240565612455276,
-0.36511551005344));
#26241=CARTESIAN_POINT('Ctrl Pts',(-0.12038866893656,-0.137966392504705,
-0.354156945213007));
#26242=CARTESIAN_POINT('Ctrl Pts',(0.0481126911101254,-0.176504221035079,
-0.343198380372572));
#26243=CARTESIAN_POINT('Ctrl Pts',(0.173623780493455,-0.0578082499262578,
-0.332239815532139));
#26244=CARTESIAN_POINT('Ctrl Pts',(0.144299756757966,0.112561276791376,
-0.321281250691706));
#26245=CARTESIAN_POINT('Ctrl Pts',(-0.0137605119892857,0.182468951639323,
-0.310322685851272));
#26246=CARTESIAN_POINT('Ctrl Pts',(-0.159535841690899,0.0896428544271446,
-0.299364121010838));
#26247=CARTESIAN_POINT('Ctrl Pts',(-0.16300976830989,-0.0831606703158766,
-0.288405556170405));
#26248=CARTESIAN_POINT('Ctrl Pts',(-0.0210751700234872,-0.18177629230341,
-0.277446991329971));
#26249=CARTESIAN_POINT('Ctrl Pts',(0.139657098315878,-0.118250656963312,
-0.266488426489538));
#26250=CARTESIAN_POINT('Ctrl Pts',(0.175815216176257,0.0507574671503514,
-0.255529861649104));
#26251=CARTESIAN_POINT('Ctrl Pts',(0.0551447377802041,0.174488474943397,
-0.244571296808671));
#26252=CARTESIAN_POINT('Ctrl Pts',(-0.114714952384342,0.14257536696912,
-0.233612731968237));
#26253=CARTESIAN_POINT('Ctrl Pts',(-0.182248350055914,-0.0165161103770323,
-0.222654167127804));
#26254=CARTESIAN_POINT('Ctrl Pts',(-0.0872151228846113,-0.160874951949878,
-0.21169560228737));
#26255=CARTESIAN_POINT('Ctrl Pts',(0.0856144901564349,-0.161732502948406,
-0.200737037446937));
#26256=CARTESIAN_POINT('Ctrl Pts',(0.182075453858757,-0.01832367121461,
-0.189778472606503));
#26257=CARTESIAN_POINT('Ctrl Pts',(0.116124144473882,0.141429933431004,
-0.178819907766069));
#26258=CARTESIAN_POINT('Ctrl Pts',(-0.0534107377320515,0.175027279764724,
-0.167861342925636));
#26259=CARTESIAN_POINT('Ctrl Pts',(-0.175302609459258,0.0524991915146761,
-0.156902778085202));
#26260=CARTESIAN_POINT('Ctrl Pts',(-0.140824166557048,-0.116858310890308,
-0.145944213244769));
#26261=CARTESIAN_POINT('Ctrl Pts',(0.0192714369799267,-0.181977841230724,
-0.134985648404336));
#26262=CARTESIAN_POINT('Ctrl Pts',(0.162174528762878,-0.0847714896391007,
-0.124027083563902));
#26263=CARTESIAN_POINT('Ctrl Pts',(0.160421360210723,0.0880503767168045,
-0.113068518723468));
#26264=CARTESIAN_POINT('Ctrl Pts',(0.0155630958780523,0.182332981603879,
-0.102109953883035));
#26265=CARTESIAN_POINT('Ctrl Pts',(-0.143161649044776,0.113969347832393,
-0.0911513890426012));
#26266=CARTESIAN_POINT('Ctrl Pts',(-0.174215737565518,-0.0560476370404291,
-0.0801928242021676));
#26267=CARTESIAN_POINT('Ctrl Pts',(-0.0498103614642923,-0.176085032876655,
-0.069234259361734));
#26268=CARTESIAN_POINT('Ctrl Pts',(0.118915079055016,-0.139024368591976,
-0.0582756945213005));
#26269=CARTESIAN_POINT('Ctrl Pts',(0.18178171708891,0.0219900978007506,
-0.0473171296808669));
#26270=CARTESIAN_POINT('Ctrl Pts',(0.0820716217526228,0.163506105608369,
-0.0363585648404334));
#26271=CARTESIAN_POINT('Ctrl Pts',(-0.0325660146575313,0.160425764828242,
-0.0290528549468111));
#26272=CARTESIAN_POINT('Ctrl Pts',(-0.0768992790589753,0.135212068175181,
-0.0253999999999999));
#26273=CARTESIAN_POINT('Ctrl Pts',(-0.0744392439309307,0.151537102412036,
-0.368404938818138));
#26274=CARTESIAN_POINT('Ctrl Pts',(-0.124125152286074,0.127130000830261,
-0.364752083871327));
#26275=CARTESIAN_POINT('Ctrl Pts',(-0.196846892776358,0.0261108931123106,
-0.357446373977704));
#26276=CARTESIAN_POINT('Ctrl Pts',(-0.13066936851252,-0.149748157727705,
-0.34648780913727));
#26277=CARTESIAN_POINT('Ctrl Pts',(0.0522213180055256,-0.191576959079111,
-0.335529244296837));
#26278=CARTESIAN_POINT('Ctrl Pts',(0.188450540704886,-0.0627448378606012,
-0.324570679456403));
#26279=CARTESIAN_POINT('Ctrl Pts',(0.156622365365713,0.12217354911568,-0.31361211461597));
#26280=CARTESIAN_POINT('Ctrl Pts',(-0.0149356033913493,0.198051053263296,
-0.302653549775536));
#26281=CARTESIAN_POINT('Ctrl Pts',(-0.173159549590572,0.0972979872867219,
-0.291694984935103));
#26282=CARTESIAN_POINT('Ctrl Pts',(-0.176930135324031,-0.0902622511839527,
-0.280736420094669));
#26283=CARTESIAN_POINT('Ctrl Pts',(-0.0228749032827522,-0.197299243655153,
-0.269777855254236));
#26284=CARTESIAN_POINT('Ctrl Pts',(0.151583242895087,-0.128348779067647,
-0.258819290413802));
#26285=CARTESIAN_POINT('Ctrl Pts',(0.190829116025446,0.0550919470945095,
-0.247860725573369));
#26286=CARTESIAN_POINT('Ctrl Pts',(0.0598538726790387,0.189389076521656,
-0.236902160732935));
#26287=CARTESIAN_POINT('Ctrl Pts',(-0.124511139789284,0.154750719746832,
-0.225943595892502));
#26288=CARTESIAN_POINT('Ctrl Pts',(-0.197811613207586,-0.0179265186027361,
-0.214985031052068));
#26289=CARTESIAN_POINT('Ctrl Pts',(-0.0946629374071695,-0.174613014384685,
-0.204026466211635));
#26290=CARTESIAN_POINT('Ctrl Pts',(0.092925617195402,-0.175543796728528,
-0.193067901371201));
#26291=CARTESIAN_POINT('Ctrl Pts',(0.197623952382857,-0.0198884377374904,
-0.182109336530767));
#26292=CARTESIAN_POINT('Ctrl Pts',(0.126040671115443,0.153507470872824,
-0.171150771690334));
#26293=CARTESIAN_POINT('Ctrl Pts',(-0.0579717961240417,0.189973893069395,
-0.1601922068499));
#26294=CARTESIAN_POINT('Ctrl Pts',(-0.190272734792916,0.0569824075906642,
-0.149233642009467));
#26295=CARTESIAN_POINT('Ctrl Pts',(-0.152849973987239,-0.126837532338885,
-0.138275077169033));
#26296=CARTESIAN_POINT('Ctrl Pts',(0.0209171388199568,-0.197518004035919,
-0.1273165123286));
#26297=CARTESIAN_POINT('Ctrl Pts',(0.176023569738343,-0.0920106278842914,
-0.116357947488166));
#26298=CARTESIAN_POINT('Ctrl Pts',(0.174120687767559,0.0955695184979354,
-0.105399382647733));
#26299=CARTESIAN_POINT('Ctrl Pts',(0.0168921205662348,0.197903471943351,
-0.0944408178072992));
#26300=CARTESIAN_POINT('Ctrl Pts',(-0.155387067912095,0.123701863660361,
-0.0834822529668656));
#26301=CARTESIAN_POINT('Ctrl Pts',(-0.18909304848802,-0.0608338758405172,
-0.0725236881264321));
#26302=CARTESIAN_POINT('Ctrl Pts',(-0.0540639624593679,-0.191121973967697,
-0.0615651232859985));
#26303=CARTESIAN_POINT('Ctrl Pts',(0.129069940086501,-0.150896480642528,
-0.050606558445565));
#26304=CARTESIAN_POINT('Ctrl Pts',(0.197305131695131,0.0238679621473913,
-0.0396479936051314));
#26305=CARTESIAN_POINT('Ctrl Pts',(0.0890802023308762,0.17746885779629,
-0.0286894287646979));
#26306=CARTESIAN_POINT('Ctrl Pts',(-0.0353470190164783,0.174125468521385,
-0.0213837188710755));
#26307=CARTESIAN_POINT('Ctrl Pts',(-0.0834661627416072,0.146758625373897,
-0.0177308639242643));
#26308=CARTESIAN_POINT('Ctrl Pts',(-0.0802959149489911,0.163459616787395,
-0.360735802742402));
#26309=CARTESIAN_POINT('Ctrl Pts',(-0.1338909712764,0.137132232879789,-0.357082947795591));
#26310=CARTESIAN_POINT('Ctrl Pts',(-0.212334254429148,0.0281652249790934,
-0.349777237901969));
#26311=CARTESIAN_POINT('Ctrl Pts',(-0.140950068088481,-0.161529922950703,
-0.338818673061535));
#26312=CARTESIAN_POINT('Ctrl Pts',(0.0563299449009258,-0.206649697123144,
-0.327860108221102));
#26313=CARTESIAN_POINT('Ctrl Pts',(0.203277300916317,-0.0676814257949445,
-0.316901543380668));
#26314=CARTESIAN_POINT('Ctrl Pts',(0.168944973973459,0.131785821439984,
-0.305942978540234));
#26315=CARTESIAN_POINT('Ctrl Pts',(-0.016110694793413,0.213633154887269,
-0.294984413699801));
#26316=CARTESIAN_POINT('Ctrl Pts',(-0.186783257490245,0.104953120146299,
-0.284025848859367));
#26317=CARTESIAN_POINT('Ctrl Pts',(-0.190850502338172,-0.0973638320520286,
-0.273067284018934));
#26318=CARTESIAN_POINT('Ctrl Pts',(-0.0246746365420171,-0.212822195006897,
-0.2621087191785));
#26319=CARTESIAN_POINT('Ctrl Pts',(0.163509387474296,-0.138446901171982,
-0.251150154338067));
#26320=CARTESIAN_POINT('Ctrl Pts',(0.205843015874634,0.0594264270386681,
-0.240191589497633));
#26321=CARTESIAN_POINT('Ctrl Pts',(0.0645630075778731,0.204289678099914,
-0.2292330246572));
#26322=CARTESIAN_POINT('Ctrl Pts',(-0.134307327194226,0.166926072524544,
-0.218274459816766));
#26323=CARTESIAN_POINT('Ctrl Pts',(-0.213374876359259,-0.0193369268284401,
-0.207315894976333));
#26324=CARTESIAN_POINT('Ctrl Pts',(-0.102110751929727,-0.188351076819492,
-0.196357330135899));
#26325=CARTESIAN_POINT('Ctrl Pts',(0.100236744234369,-0.18935509050865,
-0.185398765295466));
#26326=CARTESIAN_POINT('Ctrl Pts',(0.213172450906958,-0.0214532042603709,
-0.174440200455032));
#26327=CARTESIAN_POINT('Ctrl Pts',(0.135957197757003,0.165585008314644,
-0.163481635614599));
#26328=CARTESIAN_POINT('Ctrl Pts',(-0.062532854516032,0.204920506374065,
-0.152523070774164));
#26329=CARTESIAN_POINT('Ctrl Pts',(-0.205242860126574,0.0614656236666522,
-0.141564505933732));
#26330=CARTESIAN_POINT('Ctrl Pts',(-0.164875781417429,-0.136816753787463,
-0.130605941093298));
#26331=CARTESIAN_POINT('Ctrl Pts',(0.0225628406599869,-0.213058166841115,
-0.119647376252864));
#26332=CARTESIAN_POINT('Ctrl Pts',(0.189872610713808,-0.0992497661294819,
-0.108688811412431));
#26333=CARTESIAN_POINT('Ctrl Pts',(0.187820015324394,0.103088660279066,
-0.0977302465719972));
#26334=CARTESIAN_POINT('Ctrl Pts',(0.0182211452544175,0.213473962282823,
-0.0867716817315636));
#26335=CARTESIAN_POINT('Ctrl Pts',(-0.167612486779414,0.133434379488328,
-0.0758131168911301));
#26336=CARTESIAN_POINT('Ctrl Pts',(-0.203970359410523,-0.0656201146406053,
-0.0648545520506966));
#26337=CARTESIAN_POINT('Ctrl Pts',(-0.0583175634544437,-0.206158915058739,
-0.0538959872102629));
#26338=CARTESIAN_POINT('Ctrl Pts',(0.139224801117986,-0.162768592693081,
-0.0429374223698294));
#26339=CARTESIAN_POINT('Ctrl Pts',(0.212828546301352,0.025745826494032,
-0.0319788575293959));
#26340=CARTESIAN_POINT('Ctrl Pts',(0.0960887829091298,0.191431609984211,
-0.0210202926889623));
#26341=CARTESIAN_POINT('Ctrl Pts',(-0.0381280233754254,0.187825172214529,
-0.01371458279534));
#26342=CARTESIAN_POINT('Ctrl Pts',(-0.090033046424239,0.158305182572614,
-0.0100617278485288));
#26343=CARTESIAN_POINT('Ctrl Pts',(-0.0861525859670515,0.175382131162755,
-0.353066666666667));
#26344=CARTESIAN_POINT('Ctrl Pts',(-0.143656790266726,0.147134464929317,
-0.349413811719856));
#26345=CARTESIAN_POINT('Ctrl Pts',(-0.227821616081937,0.0302195568458765,
-0.342108101826233));
#26346=CARTESIAN_POINT('Ctrl Pts',(-0.151230767664441,-0.173311688173703,
-0.3311495369858));
#26347=CARTESIAN_POINT('Ctrl Pts',(0.0604385717963258,-0.221722435167177,
-0.320190972145366));
#26348=CARTESIAN_POINT('Ctrl Pts',(0.218104061127748,-0.072618013729288,
-0.309232407304933));
#26349=CARTESIAN_POINT('Ctrl Pts',(0.181267582581206,0.141398093764287,
-0.298273842464499));
#26350=CARTESIAN_POINT('Ctrl Pts',(-0.0172857861954766,0.229215256511242,
-0.287315277624066));
#26351=CARTESIAN_POINT('Ctrl Pts',(-0.200406965389918,0.112608253005876,
-0.276356712783632));
#26352=CARTESIAN_POINT('Ctrl Pts',(-0.204770869352314,-0.104465412920104,
-0.265398147943198));
#26353=CARTESIAN_POINT('Ctrl Pts',(-0.0264743698012821,-0.22834514635864,
-0.254439583102765));
#26354=CARTESIAN_POINT('Ctrl Pts',(0.175435532053505,-0.148545023276317,
-0.243481018262331));
#26355=CARTESIAN_POINT('Ctrl Pts',(0.220856915723823,0.0637609069828263,
-0.232522453421897));
#26356=CARTESIAN_POINT('Ctrl Pts',(0.0692721424767077,0.219190279678173,
-0.221563888581465));
#26357=CARTESIAN_POINT('Ctrl Pts',(-0.144103514599168,0.179101425302256,
-0.21060532374103));
#26358=CARTESIAN_POINT('Ctrl Pts',(-0.228938139510932,-0.0207473350541439,
-0.199646758900597));
#26359=CARTESIAN_POINT('Ctrl Pts',(-0.109558566452286,-0.202089139254299,
-0.188688194060163));
#26360=CARTESIAN_POINT('Ctrl Pts',(0.107547871273336,-0.203166384288772,
-0.17772962921973));
#26361=CARTESIAN_POINT('Ctrl Pts',(0.228720949431058,-0.0230179707832516,
-0.166771064379296));
#26362=CARTESIAN_POINT('Ctrl Pts',(0.145873724398564,0.177662545756465,
-0.155812499538863));
#26363=CARTESIAN_POINT('Ctrl Pts',(-0.0670939129080224,0.219867119678735,
-0.144853934698429));
#26364=CARTESIAN_POINT('Ctrl Pts',(-0.220212985460232,0.0659488397426404,
-0.133895369857996));
#26365=CARTESIAN_POINT('Ctrl Pts',(-0.17690158884762,-0.146795975236041,
-0.122936805017562));
#26366=CARTESIAN_POINT('Ctrl Pts',(0.024208542500017,-0.22859832964631,
-0.111978240177129));
#26367=CARTESIAN_POINT('Ctrl Pts',(0.203721651689273,-0.106488904374672,
-0.101019675336695));
#26368=CARTESIAN_POINT('Ctrl Pts',(0.20151934288123,0.110607802060197,-0.0900611104962616));
#26369=CARTESIAN_POINT('Ctrl Pts',(0.0195501699426001,0.229044452622295,
-0.079102545655828));
#26370=CARTESIAN_POINT('Ctrl Pts',(-0.179837905646733,0.143166895316295,
-0.0681439808153946));
#26371=CARTESIAN_POINT('Ctrl Pts',(-0.218847670333026,-0.0704063534406933,
-0.0571854159749609));
#26372=CARTESIAN_POINT('Ctrl Pts',(-0.0625711644495193,-0.221195856149781,
-0.0462268511345275));
#26373=CARTESIAN_POINT('Ctrl Pts',(0.149379662149471,-0.174640704743633,
-0.0352682862940938));
#26374=CARTESIAN_POINT('Ctrl Pts',(0.228351960907573,0.0276236908406728,
-0.0243097214536604));
#26375=CARTESIAN_POINT('Ctrl Pts',(0.103097363487383,0.205394362172133,
-0.0133511566132268));
#26376=CARTESIAN_POINT('Ctrl Pts',(-0.0409090277343724,0.201524875907672,
-0.00604544671960447));
#26377=CARTESIAN_POINT('Ctrl Pts',(-0.0965999301068709,0.16985173977133,
-0.00239259177279327));
#26378=CARTESIAN_POINT('Ctrl Pts',(-0.195260766042512,-0.000146819403851512,
-0.0606536358790897));
#26379=CARTESIAN_POINT('Ctrl Pts',(-0.195410942435055,-0.0204558658761102,
-0.0594975625777135));
#26380=CARTESIAN_POINT('Ctrl Pts',(-0.192485483346375,-0.0407231797866054,
-0.0583414892763372));
#26381=CARTESIAN_POINT('Ctrl Pts',(-0.186299958571393,-0.0599423957660427,
-0.057185415974961));
#26382=CARTESIAN_POINT('Ctrl Pts',(-0.16675550170519,-0.120669521010389,
-0.0535325610281498));
#26383=CARTESIAN_POINT('Ctrl Pts',(-0.114663333077355,-0.170932688580085,
-0.0498797060813386));
#26384=CARTESIAN_POINT('Ctrl Pts',(-0.0532921109969387,-0.188305080463908,
-0.0462268511345274));
#26385=CARTESIAN_POINT('Ctrl Pts',(0.00807911108347766,-0.205677472347732,
-0.0425739961877162));
#26386=CARTESIAN_POINT('Ctrl Pts',(0.0787293866164743,-0.190159088545682,
-0.038921141240905));
#26387=CARTESIAN_POINT('Ctrl Pts',(0.12721657417599,-0.148689164047273,
-0.0352682862940938));
#26388=CARTESIAN_POINT('Ctrl Pts',(0.170879723082794,-0.11134512370042,
-0.0319788575293959));
#26389=CARTESIAN_POINT('Ctrl Pts',(0.196570459065126,-0.0529565517441027,
-0.0286894287646979));
#26390=CARTESIAN_POINT('Ctrl Pts',(0.1956174094926,0.00454472201517893,
-0.0254));
#26391=CARTESIAN_POINT('',(-0.090544221732454,-0.126745838915641,-0.353066666666667));
#26392=CARTESIAN_POINT('Ctrl Pts',(-0.0905442217324535,-0.126745838915641,
-0.353066666666667));
#26393=CARTESIAN_POINT('Ctrl Pts',(-0.0950778866087321,-0.124328949845596,
-0.353066666666667));
#26394=CARTESIAN_POINT('Ctrl Pts',(-0.0994734168556016,-0.121682361637407,
-0.353066666666667));
#26395=CARTESIAN_POINT('Ctrl Pts',(-0.103710894594221,-0.118810629553691,
-0.353066666666667));
#26396=CARTESIAN_POINT('Ctrl Pts',(-0.109205802656033,-0.115086738892423,
-0.353066666666667));
#26397=CARTESIAN_POINT('Ctrl Pts',(-0.114435163201789,-0.110984556163928,
-0.353066666666667));
#26398=CARTESIAN_POINT('Ctrl Pts',(-0.119388306282607,-0.106547282912304,
-0.353066666666667));
#26399=CARTESIAN_POINT('Ctrl Pts',(-0.123142837628399,-0.103183785988989,
-0.353066666666667));
#26400=CARTESIAN_POINT('Ctrl Pts',(-0.126739923081413,-0.0996253876790819,
-0.353066666666667));
#26401=CARTESIAN_POINT('Ctrl Pts',(-0.130158509803707,-0.0959070026082769,
-0.353066666666667));
#26402=CARTESIAN_POINT('Ctrl Pts',(-0.136612470751906,-0.0888870513866671,
-0.353066666666667));
#26403=CARTESIAN_POINT('Ctrl Pts',(-0.142444637276161,-0.0812874705536567,
-0.353066666666667));
#26404=CARTESIAN_POINT('Ctrl Pts',(-0.147621095756717,-0.0732245560109258,
-0.353066666666667));
#26405=CARTESIAN_POINT('Ctrl Pts',(-0.150106918494648,-0.0693526083502609,
-0.353066666666667));
#26406=CARTESIAN_POINT('Ctrl Pts',(-0.152441921172652,-0.0653713975830042,
-0.353066666666667));
#26407=CARTESIAN_POINT('Ctrl Pts',(-0.15461137646505,-0.0613127594075525,
-0.353066666666667));
#26408=CARTESIAN_POINT('Ctrl Pts',(-0.160121027420107,-0.051005250523656,
-0.353066666666667));
#26409=CARTESIAN_POINT('Ctrl Pts',(-0.164583123630244,-0.0401759575950903,
-0.353066666666667));
#26410=CARTESIAN_POINT('Ctrl Pts',(-0.167935657633854,-0.0290196273550922,
-0.353066666666667));
#26411=CARTESIAN_POINT('Ctrl Pts',(-0.169467297684012,-0.0239227417783969,
-0.353066666666667));
#26412=CARTESIAN_POINT('Ctrl Pts',(-0.17076686879121,-0.0187570404330206,
-0.353066666666667));
#26413=CARTESIAN_POINT('Ctrl Pts',(-0.171825572631564,-0.0135389836432372,
-0.353066666666667));
#26414=CARTESIAN_POINT('Ctrl Pts',(-0.172751335094915,-0.00897615792797176,
-0.353066666666667));
#26415=CARTESIAN_POINT('Ctrl Pts',(-0.17349296837949,-0.00436905326050375,
-0.353066666666667));
#26416=CARTESIAN_POINT('Ctrl Pts',(-0.174041123319537,0.000243481210159243,
-0.353066666666667));
#26417=CARTESIAN_POINT('Ctrl Pts',(-0.174943147920424,0.00783370663915697,
-0.353066666666667));
#26418=CARTESIAN_POINT('Ctrl Pts',(-0.175325250731135,0.0154515874573274,
-0.353066666666667));
#26419=CARTESIAN_POINT('Ctrl Pts',(-0.175168987402103,0.0230468219305827,
-0.353066666666667));
#26420=CARTESIAN_POINT('Ctrl Pts',(-0.175008803924067,0.0308325966350812,
-0.353066666666667));
#26421=CARTESIAN_POINT('Ctrl Pts',(-0.174283139083255,0.0385947856858029,
-0.353066666666667));
#26422=CARTESIAN_POINT('Ctrl Pts',(-0.173027913924886,0.0462932377413482,
-0.353066666666667));
#26423=CARTESIAN_POINT('Ctrl Pts',(-0.172329203404992,0.0505785162845987,
-0.353066666666667));
#26424=CARTESIAN_POINT('Ctrl Pts',(-0.171466216089777,0.0548440796465449,
-0.353066666666667));
#26425=CARTESIAN_POINT('Ctrl Pts',(-0.170443770858798,0.0590830450887544,
-0.353066666666667));
#26426=CARTESIAN_POINT('Ctrl Pts',(-0.169609721657169,0.0625409376346687,
-0.353066666666667));
#26427=CARTESIAN_POINT('Ctrl Pts',(-0.168670590048696,0.0659761408646361,
-0.353066666666667));
#26428=CARTESIAN_POINT('Ctrl Pts',(-0.167632215380544,0.0693775142202088,
-0.353066666666667));
#26429=CARTESIAN_POINT('Ctrl Pts',(-0.164320261147807,0.0802263852757378,
-0.353066666666667));
#26430=CARTESIAN_POINT('Ctrl Pts',(-0.159996262524131,0.0907540317964261,
-0.353066666666667));
#26431=CARTESIAN_POINT('Ctrl Pts',(-0.154765649419082,0.100842798226835,
-0.353066666666667));
#26432=CARTESIAN_POINT('Ctrl Pts',(-0.151244749192667,0.107633883572982,
-0.353066666666667));
#26433=CARTESIAN_POINT('Ctrl Pts',(-0.147312170821561,0.114226277258753,
-0.353066666666667));
#26434=CARTESIAN_POINT('Ctrl Pts',(-0.142990633106768,0.120582557101035,
-0.353066666666667));
#26435=CARTESIAN_POINT('Ctrl Pts',(-0.140763809064083,0.123857853467507,
-0.353066666666667));
#26436=CARTESIAN_POINT('Ctrl Pts',(-0.138432060381342,0.127072002597403,
-0.353066666666667));
#26437=CARTESIAN_POINT('Ctrl Pts',(-0.136009717220075,0.130205302389434,
-0.353066666666667));
#26438=CARTESIAN_POINT('Ctrl Pts',(-0.128162696792256,0.140355419791331,
-0.353066666666667));
#26439=CARTESIAN_POINT('Ctrl Pts',(-0.119348186315525,0.149691156683439,
-0.353066666666667));
#26440=CARTESIAN_POINT('Ctrl Pts',(-0.109686793021438,0.158050862960414,
-0.353066666666667));
#26441=CARTESIAN_POINT('Ctrl Pts',(-0.102323091479692,0.164422447278171,
-0.353066666666667));
#26442=CARTESIAN_POINT('Ctrl Pts',(-0.0944662156361962,0.170227170930749,
-0.353066666666667));
#26443=CARTESIAN_POINT('Ctrl Pts',(-0.0861525859670518,0.175382131162755,
-0.353066666666667));
#26444=CARTESIAN_POINT('Ctrl Pts',(-0.0905442217324539,-0.126745838915641,
-0.353066666666667));
#26445=CARTESIAN_POINT('Ctrl Pts',(-0.0531162262373072,-0.153109051305698,
-0.349777237901969));
#26446=CARTESIAN_POINT('Ctrl Pts',(0.0522750989337435,-0.172567827516364,
-0.342834954190459));
#26447=CARTESIAN_POINT('Ctrl Pts',(0.173623780493455,-0.0578082499262578,
-0.332239815532139));
#26448=CARTESIAN_POINT('Ctrl Pts',(0.144299756757966,0.112561276791376,
-0.321281250691706));
#26449=CARTESIAN_POINT('Ctrl Pts',(-0.0137605119892857,0.182468951639323,
-0.310322685851272));
#26450=CARTESIAN_POINT('Ctrl Pts',(-0.136232288784936,0.104481976189832,
-0.301115950322802));
#26451=CARTESIAN_POINT('Ctrl Pts',(-0.155286340637538,0.0266232940100586,
-0.295562069741144));
#26452=CARTESIAN_POINT('Ctrl Pts',(-0.15531185862521,-1.5337286706104E-5,
-0.293661044106296));
#26453=CARTESIAN_POINT('Origin',(-2.59090492670967E-17,0.,-0.353066666666667));
#26454=CARTESIAN_POINT('',(-0.1954,-2.39295984553393E-17,-0.353066666666667));
#26455=CARTESIAN_POINT('Origin',(0.,0.,-0.353066666666667));
#26456=CARTESIAN_POINT('Origin',(0.,0.,-0.353066666666667));
#26457=CARTESIAN_POINT('',(0.090360677865019,-0.126612599672285,-0.353066666666667));
#26458=CARTESIAN_POINT('Ctrl Pts',(0.0863529496556134,0.175584683415656,
-0.353066666666667));
#26459=CARTESIAN_POINT('Ctrl Pts',(0.091775925641401,0.172264613803354,
-0.353066666666667));
#26460=CARTESIAN_POINT('Ctrl Pts',(0.0970151064363841,0.168672722682513,
-0.353066666666667));
#26461=CARTESIAN_POINT('Ctrl Pts',(0.102046076702462,0.164808456407418,
-0.353066666666667));
#26462=CARTESIAN_POINT('Ctrl Pts',(0.109748329747439,0.158892389503854,
-0.353066666666667));
#26463=CARTESIAN_POINT('Ctrl Pts',(0.11696333598913,0.152338121455057,-0.353066666666667));
#26464=CARTESIAN_POINT('Ctrl Pts',(0.123648657619329,0.145228304456469,
-0.353066666666667));
#26465=CARTESIAN_POINT('Ctrl Pts',(0.126392710732544,0.14231001322853,-0.353066666666667));
#26466=CARTESIAN_POINT('Ctrl Pts',(0.129045803306702,0.139299406002297,
-0.353066666666667));
#26467=CARTESIAN_POINT('Ctrl Pts',(0.131599361332803,0.136209297313463,
-0.353066666666667));
#26468=CARTESIAN_POINT('Ctrl Pts',(0.136248057252147,0.130583822777432,
-0.353066666666667));
#26469=CARTESIAN_POINT('Ctrl Pts',(0.140573104671842,0.124688829108862,
-0.353066666666667));
#26470=CARTESIAN_POINT('Ctrl Pts',(0.144556667852106,0.118560041485065,
-0.353066666666667));
#26471=CARTESIAN_POINT('Ctrl Pts',(0.147882589890062,0.113443047251125,
-0.353066666666667));
#26472=CARTESIAN_POINT('Ctrl Pts',(0.150970393632736,0.108162994083143,
-0.353066666666667));
#26473=CARTESIAN_POINT('Ctrl Pts',(0.153806693424657,0.102740045379718,
-0.353066666666667));
#26474=CARTESIAN_POINT('Ctrl Pts',(0.155695835469646,0.0991280434211665,
-0.353066666666667));
#26475=CARTESIAN_POINT('Ctrl Pts',(0.157468792252594,0.0954612486662374,
-0.353066666666667));
#26476=CARTESIAN_POINT('Ctrl Pts',(0.159121858455566,0.0917483027491353,
-0.353066666666667));
#26477=CARTESIAN_POINT('Ctrl Pts',(0.164086071592859,0.0805982018840912,
-0.353066666666667));
#26478=CARTESIAN_POINT('Ctrl Pts',(0.167976354467203,0.0690254035666524,
-0.353066666666667));
#26479=CARTESIAN_POINT('Ctrl Pts',(0.170691731659898,0.0571968233482779,
-0.353066666666667));
#26480=CARTESIAN_POINT('Ctrl Pts',(0.171976315344167,0.0516009889288562,
-0.353066666666667));
#26481=CARTESIAN_POINT('Ctrl Pts',(0.172997217266348,0.0459478680695661,
-0.353066666666667));
#26482=CARTESIAN_POINT('Ctrl Pts',(0.173739546526888,0.0402557306321508,
-0.353066666666667));
#26483=CARTESIAN_POINT('Ctrl Pts',(0.174228988637866,0.0365027170956556,
-0.353066666666667));
#26484=CARTESIAN_POINT('Ctrl Pts',(0.174597145890101,0.0327307795264523,
-0.353066666666667));
#26485=CARTESIAN_POINT('Ctrl Pts',(0.174838710766854,0.0289627049718209,
-0.353066666666667));
#26486=CARTESIAN_POINT('Ctrl Pts',(0.175337568406377,0.0211812228162318,
-0.353066666666667));
#26487=CARTESIAN_POINT('Ctrl Pts',(0.175299889017541,0.0134005598576949,
-0.353066666666667));
#26488=CARTESIAN_POINT('Ctrl Pts',(0.174695429084084,0.00566655864109738,
-0.353066666666667));
#26489=CARTESIAN_POINT('Ctrl Pts',(0.1741598428623,-0.00118621068504322,
-0.353066666666667));
#26490=CARTESIAN_POINT('Ctrl Pts',(0.173179021113242,-0.00800243245789652,
-0.353066666666667));
#26491=CARTESIAN_POINT('Ctrl Pts',(0.171772005196112,-0.0147481282838624,
-0.353066666666667));
#26492=CARTESIAN_POINT('Ctrl Pts',(0.170726249047483,-0.0197618262818046,
-0.353066666666667));
#26493=CARTESIAN_POINT('Ctrl Pts',(0.169444930850078,-0.0247365274644173,
-0.353066666666667));
#26494=CARTESIAN_POINT('Ctrl Pts',(0.167934206696833,-0.0296569328335628,
-0.353066666666667));
#26495=CARTESIAN_POINT('Ctrl Pts',(0.166832256855383,-0.0332459665461353,
-0.353066666666667));
#26496=CARTESIAN_POINT('Ctrl Pts',(0.165610219623287,-0.0367990811940273,
-0.353066666666667));
#26497=CARTESIAN_POINT('Ctrl Pts',(0.164274304450244,-0.0403041213275535,
-0.353066666666667));
#26498=CARTESIAN_POINT('Ctrl Pts',(0.160829473997209,-0.0493423216824256,
-0.353066666666667));
#26499=CARTESIAN_POINT('Ctrl Pts',(0.156624378199029,-0.0580767247737816,
-0.353066666666667));
#26500=CARTESIAN_POINT('Ctrl Pts',(0.151713593210745,-0.0664101273423615,
-0.353066666666667));
#26501=CARTESIAN_POINT('Ctrl Pts',(0.148533489359529,-0.0718066343499594,
-0.353066666666667));
#26502=CARTESIAN_POINT('Ctrl Pts',(0.145056996731404,-0.0770347033166309,
-0.353066666666667));
#26503=CARTESIAN_POINT('Ctrl Pts',(0.141295320169661,-0.082063260429383,
-0.353066666666667));
#26504=CARTESIAN_POINT('Ctrl Pts',(0.138558394341238,-0.0857219449589262,
-0.353066666666667));
#26505=CARTESIAN_POINT('Ctrl Pts',(0.135667276928843,-0.0892779006893289,
-0.353066666666667));
#26506=CARTESIAN_POINT('Ctrl Pts',(0.13264496147214,-0.0926975714274839,
-0.353066666666667));
#26507=CARTESIAN_POINT('Ctrl Pts',(0.125506731853708,-0.100774291180298,
-0.353066666666667));
#26508=CARTESIAN_POINT('Ctrl Pts',(0.117622588801953,-0.108117960820719,
-0.353066666666667));
#26509=CARTESIAN_POINT('Ctrl Pts',(0.109058683323211,-0.1145742204159,-0.353066666666667));
#26510=CARTESIAN_POINT('Ctrl Pts',(0.103144935763732,-0.119032547229425,
-0.353066666666667));
#26511=CARTESIAN_POINT('Ctrl Pts',(0.0969064199016059,-0.123066975878573,
-0.353066666666667));
#26512=CARTESIAN_POINT('Ctrl Pts',(0.0903606778650195,-0.126612599672284,
-0.353066666666667));
#26513=CARTESIAN_POINT('Origin',(0.,0.,-0.353066666666667));
#26514=CARTESIAN_POINT('Origin',(0.,0.,-0.482472289227037));
#26515=CARTESIAN_POINT('Ctrl Pts',(0.090360677865019,-0.126612599672285,
-0.353066666666667));
#26516=CARTESIAN_POINT('Ctrl Pts',(0.131874352891076,-0.0969851863995775,
-0.349413811719856));
#26517=CARTESIAN_POINT('Ctrl Pts',(0.182857874798175,0.00573779165809946,
-0.342108101826233));
#26518=CARTESIAN_POINT('Ctrl Pts',(0.0963663073753999,0.155697320567796,
-0.3311495369858));
#26519=CARTESIAN_POINT('Ctrl Pts',(-0.0761582306436912,0.166338694028791,
-0.320190972145365));
#26520=CARTESIAN_POINT('Ctrl Pts',(-0.151457270014338,0.0672989293663021,
-0.312298556225779));
#26521=CARTESIAN_POINT('Ctrl Pts',(-0.155721140989265,0.00830051131805939,
-0.308058995253002));
#26522=CARTESIAN_POINT('Ctrl Pts',(-0.155653088469525,0.000125523659554115,
-0.307472289227037));
#26523=CARTESIAN_POINT('Ctrl Pts',(0.113509973994373,-0.159049193030951,
-0.376074074893873));
#26524=CARTESIAN_POINT('Ctrl Pts',(0.165658942815277,-0.121831600273079,
-0.372421219947062));
#26525=CARTESIAN_POINT('Ctrl Pts',(0.229703817007801,0.00720774342650353,
-0.365115510053439));
#26526=CARTESIAN_POINT('Ctrl Pts',(0.121054172042129,0.195585062288314,
-0.354156945213007));
#26527=CARTESIAN_POINT('Ctrl Pts',(-0.0956690341869317,0.208952624964486,
-0.343198380372572));
#26528=CARTESIAN_POINT('Ctrl Pts',(-0.22700621729006,0.0362066800668334,
-0.332239815532139));
#26529=CARTESIAN_POINT('Ctrl Pts',(-0.15587805676934,-0.168977471396189,
-0.321281250691706));
#26530=CARTESIAN_POINT('Ctrl Pts',(0.0543075797275565,-0.223358798671181,
-0.310322685851272));
#26531=CARTESIAN_POINT('Ctrl Pts',(0.216043556493043,-0.0785414608874288,
-0.299364121010839));
#26532=CARTESIAN_POINT('Ctrl Pts',(0.185071090564807,0.136355543216117,
-0.288405556170405));
#26533=CARTESIAN_POINT('Ctrl Pts',(-0.0109877667305077,0.229612032449797,
-0.277446991329971));
#26534=CARTESIAN_POINT('Ctrl Pts',(-0.197244472898579,0.118058803257178,
-0.266488426489538));
#26535=CARTESIAN_POINT('Ctrl Pts',(-0.207558494710389,-0.0988064563337987,
-0.255529861649104));
#26536=CARTESIAN_POINT('Ctrl Pts',(-0.0327288714983575,-0.227534271296709,
-0.244571296808671));
#26537=CARTESIAN_POINT('Ctrl Pts',(0.171294954925333,-0.153300998465301,
-0.233612731968237));
#26538=CARTESIAN_POINT('Ctrl Pts',(0.222522760696156,0.0576780642727636,
-0.222654167127804));
#26539=CARTESIAN_POINT('Ctrl Pts',(0.0752589587035167,0.217207742637096,
-0.21169560228737));
#26540=CARTESIAN_POINT('Ctrl Pts',(-0.139136279132604,0.182986979233611,
-0.200737037446937));
#26541=CARTESIAN_POINT('Ctrl Pts',(-0.229421104700159,-0.0144592892217846,
-0.189778472606503));
#26542=CARTESIAN_POINT('Ctrl Pts',(-0.115061091986856,-0.19900774667556,
-0.178819907766069));
#26543=CARTESIAN_POINT('Ctrl Pts',(0.101934294664377,-0.206040183664755,
-0.167861342925636));
#26544=CARTESIAN_POINT('Ctrl Pts',(0.228003284630101,-0.0292835421690294,
-0.156902778085202));
#26545=CARTESIAN_POINT('Ctrl Pts',(0.150692832428747,0.173594109330608,
-0.145944213244769));
#26546=CARTESIAN_POINT('Ctrl Pts',(-0.0610380283237141,0.221624958463411,
-0.134985648404335));
#26547=CARTESIAN_POINT('Ctrl Pts',(-0.21831968438096,0.0719647960828687,
-0.124027083563902));
#26548=CARTESIAN_POINT('Ctrl Pts',(-0.180864527330742,-0.14188786234924,
-0.113068518723468));
#26549=CARTESIAN_POINT('Ctrl Pts',(0.0179335408659357,-0.229176716732969,
-0.102109953883035));
#26550=CARTESIAN_POINT('Ctrl Pts',(0.200714315904756,-0.112036733041374,
-0.0911513890426012));
#26551=CARTESIAN_POINT('Ctrl Pts',(0.204495895156562,0.105037056726432,
-0.0801928242021676));
#26552=CARTESIAN_POINT('Ctrl Pts',(0.0257911334986473,0.228424087614811,
-0.0692342593617342));
#26553=CARTESIAN_POINT('Ctrl Pts',(-0.175776163519519,0.148042236946653,
-0.0582756945213006));
#26554=CARTESIAN_POINT('Ctrl Pts',(-0.220826613807624,-0.0643679717979928,
-0.047317129680867));
#26555=CARTESIAN_POINT('Ctrl Pts',(-0.0683468568897243,-0.219418554973255,
-0.0363585648404335));
#26556=CARTESIAN_POINT('Ctrl Pts',(0.0731165658398347,-0.192197273548725,
-0.0290528549468112));
#26557=CARTESIAN_POINT('Ctrl Pts',(0.122919639333555,-0.151894444487311,
-0.0254));
#26558=CARTESIAN_POINT('Ctrl Pts',(0.105793541951255,-0.148236995244729,
-0.368404938818138));
#26559=CARTESIAN_POINT('Ctrl Pts',(0.154397412840543,-0.113549462315245,
-0.364752083871327));
#26560=CARTESIAN_POINT('Ctrl Pts',(0.214088502937926,0.0067177595037024,
-0.357446373977704));
#26561=CARTESIAN_POINT('Ctrl Pts',(0.112824883819886,0.182289148381474,
-0.346487809137271));
#26562=CARTESIAN_POINT('Ctrl Pts',(-0.0891654330058515,0.194747981319255,
-0.335529244296837));
#26563=CARTESIAN_POINT('Ctrl Pts',(-0.211574286619625,0.033745342297022,
-0.324570679456403));
#26564=CARTESIAN_POINT('Ctrl Pts',(-0.145281433496979,-0.15749034714655,
-0.313612114615971));
#26565=CARTESIAN_POINT('Ctrl Pts',(0.0506157389698917,-0.208174820290003,
-0.302653549775536));
#26566=CARTESIAN_POINT('Ctrl Pts',(0.201356869822541,-0.0732021957622769,
-0.291694984935103));
#26567=CARTESIAN_POINT('Ctrl Pts',(0.172489918679772,0.127086064544738,
-0.280736420094669));
#26568=CARTESIAN_POINT('Ctrl Pts',(-0.0102408160239047,0.21400295791359,
-0.269777855254236));
#26569=CARTESIAN_POINT('Ctrl Pts',(-0.183835751907435,0.110033140838552,
-0.258819290413802));
#26570=CARTESIAN_POINT('Ctrl Pts',(-0.193448624334734,-0.0920895725315098,
-0.247860725573369));
#26571=CARTESIAN_POINT('Ctrl Pts',(-0.0305039558906986,-0.212066443403201,
-0.236902160732935));
#26572=CARTESIAN_POINT('Ctrl Pts',(0.159650287655161,-0.142879564161578,
-0.225943595892502));
#26573=CARTESIAN_POINT('Ctrl Pts',(0.207395616353369,0.0537570972627508,
-0.214985031052068));
#26574=CARTESIAN_POINT('Ctrl Pts',(0.0701428387711811,0.202441914346259,
-0.204026466211635));
#26575=CARTESIAN_POINT('Ctrl Pts',(-0.129677765445408,0.170547485677727,
-0.193067901371201));
#26576=CARTESIAN_POINT('Ctrl Pts',(-0.21382500947276,-0.0134763436818869,
-0.182109336530767));
#26577=CARTESIAN_POINT('Ctrl Pts',(-0.107239214614499,-0.185479157960068,
-0.171150771690334));
#26578=CARTESIAN_POINT('Ctrl Pts',(0.095004779750738,-0.192033528395153,
-0.1601922068499));
#26579=CARTESIAN_POINT('Ctrl Pts',(0.212503573110978,-0.0272928407779753,
-0.149233642009467));
#26580=CARTESIAN_POINT('Ctrl Pts',(0.1404487018039,0.161793145057621,-0.138275077169034));
#26581=CARTESIAN_POINT('Ctrl Pts',(-0.056888650246778,0.20655884690632,
-0.1273165123286));
#26582=CARTESIAN_POINT('Ctrl Pts',(-0.203478266055164,0.067072614022305,
-0.116357947488167));
#26583=CARTESIAN_POINT('Ctrl Pts',(-0.168569318504181,-0.132242295452929,
-0.105399382647733));
#26584=CARTESIAN_POINT('Ctrl Pts',(0.0167144149643532,-0.213597235051276,
-0.0944408178072993));
#26585=CARTESIAN_POINT('Ctrl Pts',(0.18706971425207,-0.104420452229878,
-0.0834822529668657));
#26586=CARTESIAN_POINT('Ctrl Pts',(0.190594220946413,0.0978966153914813,
-0.0725236881264321));
#26587=CARTESIAN_POINT('Ctrl Pts',(0.0240378467877621,0.212895769819775,
-0.0615651232859986));
#26588=CARTESIAN_POINT('Ctrl Pts',(-0.163826862741196,0.137978294363364,
-0.0506065584455651));
#26589=CARTESIAN_POINT('Ctrl Pts',(-0.205814773889109,-0.0599922234592858,
-0.0396479936051315));
#26590=CARTESIAN_POINT('Ctrl Pts',(-0.0637006231008205,-0.204502435192149,
-0.028689428764698));
#26591=CARTESIAN_POINT('Ctrl Pts',(0.0681460862275567,-0.179131662237028,
-0.0213837188710756));
#26592=CARTESIAN_POINT('Ctrl Pts',(0.114563536250235,-0.141568628020543,
-0.0177308639242644));
#26593=CARTESIAN_POINT('Ctrl Pts',(0.098077109908137,-0.137424797458507,
-0.360735802742402));
#26594=CARTESIAN_POINT('Ctrl Pts',(0.14313588286581,-0.105267324357411,
-0.357082947795591));
#26595=CARTESIAN_POINT('Ctrl Pts',(0.19847318886805,0.0062277755809008,
-0.349777237901968));
#26596=CARTESIAN_POINT('Ctrl Pts',(0.104595595597643,0.168993234474635,
-0.338818673061536));
#26597=CARTESIAN_POINT('Ctrl Pts',(-0.0826618318247713,0.180543337674023,
-0.327860108221101));
#26598=CARTESIAN_POINT('Ctrl Pts',(-0.19614235594919,0.031284004527211,
-0.316901543380668));
#26599=CARTESIAN_POINT('Ctrl Pts',(-0.134684810224618,-0.146003222896912,
-0.305942978540235));
#26600=CARTESIAN_POINT('Ctrl Pts',(0.0469238982122269,-0.192990841908825,
-0.294984413699801));
#26601=CARTESIAN_POINT('Ctrl Pts',(0.18667018315204,-0.0678629306371251,
-0.284025848859368));
#26602=CARTESIAN_POINT('Ctrl Pts',(0.159908746794737,0.117816585873359,
-0.273067284018934));
#26603=CARTESIAN_POINT('Ctrl Pts',(-0.00949386531730154,0.198393883377383,
-0.2621087191785));
#26604=CARTESIAN_POINT('Ctrl Pts',(-0.170427030916291,0.102007478419926,
-0.251150154338067));
#26605=CARTESIAN_POINT('Ctrl Pts',(-0.179338753959079,-0.0853726887292205,
-0.240191589497633));
#26606=CARTESIAN_POINT('Ctrl Pts',(-0.0282790402830398,-0.196598615509695,
-0.2292330246572));
#26607=CARTESIAN_POINT('Ctrl Pts',(0.14800562038499,-0.132458129857856,
-0.218274459816766));
#26608=CARTESIAN_POINT('Ctrl Pts',(0.192268472010582,0.0498361302527376,
-0.207315894976333));
#26609=CARTESIAN_POINT('Ctrl Pts',(0.0650267188388455,0.187676086055423,
-0.196357330135899));
#26610=CARTESIAN_POINT('Ctrl Pts',(-0.120219251758212,0.158107992121843,
-0.185398765295466));
#26611=CARTESIAN_POINT('Ctrl Pts',(-0.198228914245361,-0.0124933981419889,
-0.174440200455032));
#26612=CARTESIAN_POINT('Ctrl Pts',(-0.0994173372421406,-0.171950569244577,
-0.163481635614598));
#26613=CARTESIAN_POINT('Ctrl Pts',(0.0880752648370985,-0.178026873125552,
-0.152523070774165));
#26614=CARTESIAN_POINT('Ctrl Pts',(0.197003861591856,-0.0253021393869213,
-0.141564505933731));
#26615=CARTESIAN_POINT('Ctrl Pts',(0.130204571179052,0.149992180784635,
-0.130605941093298));
#26616=CARTESIAN_POINT('Ctrl Pts',(-0.0527392721698415,0.191492735349228,
-0.119647376252864));
#26617=CARTESIAN_POINT('Ctrl Pts',(-0.188636847729369,0.0621804319617416,
-0.108688811412431));
#26618=CARTESIAN_POINT('Ctrl Pts',(-0.15627410967762,-0.122596728556619,
-0.097730246571997));
#26619=CARTESIAN_POINT('Ctrl Pts',(0.015495289062771,-0.198017753369582,
-0.0867716817315639));
#26620=CARTESIAN_POINT('Ctrl Pts',(0.173425112599384,-0.0968041714183824,
-0.07581311689113));
#26621=CARTESIAN_POINT('Ctrl Pts',(0.176692546736265,0.0907561740565302,
-0.0648545520506967));
#26622=CARTESIAN_POINT('Ctrl Pts',(0.0222845600768763,0.197367452024739,
-0.053895987210263));
#26623=CARTESIAN_POINT('Ctrl Pts',(-0.151877561962873,0.127914351780075,
-0.0429374223698296));
#26624=CARTESIAN_POINT('Ctrl Pts',(-0.190802933970593,-0.0556164751205788,
-0.031978857529396));
#26625=CARTESIAN_POINT('Ctrl Pts',(-0.0590543893119163,-0.189586315411043,
-0.0210202926889625));
#26626=CARTESIAN_POINT('Ctrl Pts',(0.0631756066152784,-0.166066050925332,
-0.0137145827953401));
#26627=CARTESIAN_POINT('Ctrl Pts',(0.106207433166915,-0.131242811553775,
-0.0100617278485289));
#26628=CARTESIAN_POINT('Ctrl Pts',(0.090360677865019,-0.126612599672285,
-0.353066666666667));
#26629=CARTESIAN_POINT('Ctrl Pts',(0.131874352891076,-0.0969851863995775,
-0.349413811719856));
#26630=CARTESIAN_POINT('Ctrl Pts',(0.182857874798175,0.00573779165809946,
-0.342108101826233));
#26631=CARTESIAN_POINT('Ctrl Pts',(0.0963663073753999,0.155697320567796,
-0.3311495369858));
#26632=CARTESIAN_POINT('Ctrl Pts',(-0.0761582306436912,0.166338694028791,
-0.320190972145365));
#26633=CARTESIAN_POINT('Ctrl Pts',(-0.180710425278755,0.0288226667573998,
-0.309232407304933));
#26634=CARTESIAN_POINT('Ctrl Pts',(-0.124088186952256,-0.134516098647273,
-0.298273842464499));
#26635=CARTESIAN_POINT('Ctrl Pts',(0.0432320574545622,-0.177806863527647,
-0.287315277624065));
#26636=CARTESIAN_POINT('Ctrl Pts',(0.171983496481539,-0.0625236655119731,
-0.276356712783632));
#26637=CARTESIAN_POINT('Ctrl Pts',(0.147327574909702,0.10854710720198,-0.265398147943198));
#26638=CARTESIAN_POINT('Ctrl Pts',(-0.00874691461069841,0.182784808841176,
-0.254439583102765));
#26639=CARTESIAN_POINT('Ctrl Pts',(-0.157018309925148,0.0939818160013004,
-0.243481018262331));
#26640=CARTESIAN_POINT('Ctrl Pts',(-0.165228883583424,-0.0786558049269315,
-0.232522453421898));
#26641=CARTESIAN_POINT('Ctrl Pts',(-0.0260541246753813,-0.181130787616187,
-0.221563888581464));
#26642=CARTESIAN_POINT('Ctrl Pts',(0.136360953114818,-0.122036695554133,
-0.21060532374103));
#26643=CARTESIAN_POINT('Ctrl Pts',(0.177141327667794,0.0459151632427247,
-0.199646758900597));
#26644=CARTESIAN_POINT('Ctrl Pts',(0.0599105989065099,0.172910257764587,
-0.188688194060163));
#26645=CARTESIAN_POINT('Ctrl Pts',(-0.110760738071016,0.145668498565958,
-0.17772962921973));
#26646=CARTESIAN_POINT('Ctrl Pts',(-0.182632819017962,-0.0115104526020911,
-0.166771064379296));
#26647=CARTESIAN_POINT('Ctrl Pts',(-0.0915954598697826,-0.158421980529086,
-0.155812499538863));
#26648=CARTESIAN_POINT('Ctrl Pts',(0.081145749923459,-0.16402021785595,
-0.144853934698429));
#26649=CARTESIAN_POINT('Ctrl Pts',(0.181504150072734,-0.0233114379958674,
-0.133895369857996));
#26650=CARTESIAN_POINT('Ctrl Pts',(0.119960440554205,0.138191216511648,
-0.122936805017562));
#26651=CARTESIAN_POINT('Ctrl Pts',(-0.0485898940929054,0.176426623792137,
-0.111978240177129));
#26652=CARTESIAN_POINT('Ctrl Pts',(-0.173795429403574,0.057288249901178,
-0.101019675336695));
#26653=CARTESIAN_POINT('Ctrl Pts',(-0.143978900851059,-0.112951161660308,
-0.0900611104962616));
#26654=CARTESIAN_POINT('Ctrl Pts',(0.0142761631611888,-0.182438271687888,
-0.0791025456558283));
#26655=CARTESIAN_POINT('Ctrl Pts',(0.159780510946698,-0.0891878906068867,
-0.0681439808153946));
#26656=CARTESIAN_POINT('Ctrl Pts',(0.162790872526117,0.083615732721579,
-0.0571854159749611));
#26657=CARTESIAN_POINT('Ctrl Pts',(0.0205312733659909,0.181839134229702,
-0.0462268511345275));
#26658=CARTESIAN_POINT('Ctrl Pts',(-0.13992826118455,0.117850409196786,
-0.035268286294094));
#26659=CARTESIAN_POINT('Ctrl Pts',(-0.175791094052078,-0.051240726781872,
-0.0243097214536604));
#26660=CARTESIAN_POINT('Ctrl Pts',(-0.0544081555230124,-0.174670195629937,
-0.0133511566132269));
#26661=CARTESIAN_POINT('Ctrl Pts',(0.0582051270030004,-0.153000439613635,
-0.00604544671960458));
#26662=CARTESIAN_POINT('Ctrl Pts',(0.0978513300835948,-0.120916995087007,
-0.00239259177279338));
#26663=CARTESIAN_POINT('Ctrl Pts',(0.122919639333553,-0.151894444487312,
-0.0254000000000001));
#26664=CARTESIAN_POINT('Ctrl Pts',(0.0731165658398337,-0.192197273548725,
-0.0290528549468112));
#26665=CARTESIAN_POINT('Ctrl Pts',(0.00238485447505431,-0.20580791426099,
-0.0327057098936224));
#26666=CARTESIAN_POINT('Ctrl Pts',(-0.058394294026985,-0.186771470754579,
-0.0363585648404336));
#26667=CARTESIAN_POINT('Ctrl Pts',(-0.119173442529025,-0.167735027248167,
-0.0400114197872447));
#26668=CARTESIAN_POINT('Ctrl Pts',(-0.170000028168324,-0.11605149952308,
-0.0436642747340559));
#26669=CARTESIAN_POINT('Ctrl Pts',(-0.187904912606623,-0.0548080342030955,
-0.0473171296808671));
#26670=CARTESIAN_POINT('Ctrl Pts',(-0.193072141284385,-0.0371335838922075,
-0.0483713189386592));
#26671=CARTESIAN_POINT('Ctrl Pts',(-0.195497451170818,-0.0186629240423492,
-0.0494255081964514));
#26672=CARTESIAN_POINT('Ctrl Pts',(-0.195345140381879,-0.000154736422984442,
-0.0504796974542436));
#26673=CARTESIAN_POINT('Origin',(0.,0.,-0.199));
#26674=CARTESIAN_POINT('',(0.0577350269189626,-0.1,-0.199));
#26675=CARTESIAN_POINT('',(-0.0577350269189627,-0.1,-0.199));
#26676=CARTESIAN_POINT('',(0.0288675134594813,-0.1,-0.199));
#26677=CARTESIAN_POINT('Origin',(0.,0.,-0.199));
#26678=CARTESIAN_POINT('Origin',(0.,0.,-0.199));
#26679=CARTESIAN_POINT('',(-0.115470053837925,2.77555756156289E-17,-0.199));
#26680=CARTESIAN_POINT('',(-0.0721687836487033,-0.075,-0.199));
#26681=CARTESIAN_POINT('Origin',(0.,0.,-0.199));
#26682=CARTESIAN_POINT('Origin',(0.,0.,-0.199));
#26683=CARTESIAN_POINT('',(-0.0577350269189626,0.1,-0.199));
#26684=CARTESIAN_POINT('',(-0.101036297108185,0.025,-0.199));
#26685=CARTESIAN_POINT('Origin',(0.,0.,-0.199));
#26686=CARTESIAN_POINT('Origin',(0.,0.,-0.199));
#26687=CARTESIAN_POINT('',(0.0577350269189626,0.1,-0.199));
#26688=CARTESIAN_POINT('',(-0.0288675134594813,0.1,-0.199));
#26689=CARTESIAN_POINT('Origin',(0.,0.,-0.199));
#26690=CARTESIAN_POINT('Origin',(0.,0.,-0.199));
#26691=CARTESIAN_POINT('',(0.115470053837925,0.,-0.199));
#26692=CARTESIAN_POINT('',(0.0721687836487032,0.075,-0.199));
#26693=CARTESIAN_POINT('Origin',(0.,0.,-0.199));
#26694=CARTESIAN_POINT('Origin',(0.,0.,-0.199));
#26695=CARTESIAN_POINT('',(0.101036297108185,-0.025,-0.199));
#26696=CARTESIAN_POINT('Origin',(0.,0.,-0.199));
#26697=CARTESIAN_POINT('Origin',(0.,0.,-0.234141016151378));
#26698=CARTESIAN_POINT('',(0.,0.,-0.269282032302755));
#26699=CARTESIAN_POINT('',(-0.113827101150665,-1.39397995080384E-17,-0.2));
#26700=CARTESIAN_POINT('',(-0.0577350269189626,-7.07050159149938E-18,-0.234141016151378));
#26701=CARTESIAN_POINT('',(-0.113789894775128,-0.00291012086156119,-0.2));
#26702=CARTESIAN_POINT('Origin',(0.,0.,-0.2));
#26703=CARTESIAN_POINT('Ctrl Pts',(-0.115470053837925,-1.38777878078145E-17,
-0.199));
#26704=CARTESIAN_POINT('Ctrl Pts',(-0.114623954995367,-0.00146548618353618,
-0.199514986736453));
#26705=CARTESIAN_POINT('Ctrl Pts',(-0.113789894775128,-0.00291012086156124,
-0.2));
#26706=CARTESIAN_POINT('',(-0.0594151859817593,-0.0970898791384388,-0.2));
#26707=CARTESIAN_POINT('Ctrl Pts',(-0.0594151859817594,-0.0970898791384387,
-0.2));
#26708=CARTESIAN_POINT('Ctrl Pts',(-0.0585811257615208,-0.0985345138164641,
-0.199514986736453));
#26709=CARTESIAN_POINT('Ctrl Pts',(-0.0577350269189627,-0.1,-0.199));
#26710=CARTESIAN_POINT('',(-0.0543747087933692,-0.1,-0.2));
#26711=CARTESIAN_POINT('Origin',(0.,0.,-0.2));
#26712=CARTESIAN_POINT('Ctrl Pts',(-0.0577350269189627,-0.1,-0.199));
#26713=CARTESIAN_POINT('Ctrl Pts',(-0.0560428292338519,-0.1,-0.199514986736451));
#26714=CARTESIAN_POINT('Ctrl Pts',(-0.0543747087933692,-0.1,-0.2));
#26715=CARTESIAN_POINT('',(0.0543747087933691,-0.1,-0.2));
#26716=CARTESIAN_POINT('Ctrl Pts',(0.0543747087933691,-0.1,-0.2));
#26717=CARTESIAN_POINT('Ctrl Pts',(0.056042829233854,-0.1,-0.19951498673645));
#26718=CARTESIAN_POINT('Ctrl Pts',(0.0577350269189626,-0.1,-0.199));
#26719=CARTESIAN_POINT('',(0.0594151859817594,-0.0970898791384387,-0.2));
#26720=CARTESIAN_POINT('Origin',(0.,0.,-0.2));
#26721=CARTESIAN_POINT('Ctrl Pts',(0.0577350269189626,-0.1,-0.199));
#26722=CARTESIAN_POINT('Ctrl Pts',(0.0585811257615188,-0.0985345138164674,
-0.199514986736451));
#26723=CARTESIAN_POINT('Ctrl Pts',(0.0594151859817594,-0.0970898791384387,
-0.2));
#26724=CARTESIAN_POINT('',(0.113789894775128,-0.00291012086156127,-0.2));
#26725=CARTESIAN_POINT('Ctrl Pts',(0.113789894775128,-0.00291012086156127,
-0.2));
#26726=CARTESIAN_POINT('Ctrl Pts',(0.114623954995369,-0.00146548618353307,
-0.199514986736452));
#26727=CARTESIAN_POINT('Ctrl Pts',(0.115470053837925,1.38777878078145E-17,
-0.199));
#26728=CARTESIAN_POINT('',(0.113789894775128,0.00291012086156127,-0.2));
#26729=CARTESIAN_POINT('Origin',(0.,0.,-0.2));
#26730=CARTESIAN_POINT('Ctrl Pts',(0.115470053837925,0.,-0.199));
#26731=CARTESIAN_POINT('Ctrl Pts',(0.114623954995369,0.00146548618353293,
-0.199514986736452));
#26732=CARTESIAN_POINT('Ctrl Pts',(0.113789894775128,0.00291012086156128,
-0.2));
#26733=CARTESIAN_POINT('',(0.0594151859817593,0.0970898791384387,-0.2));
#26734=CARTESIAN_POINT('Ctrl Pts',(0.0594151859817593,0.0970898791384387,
-0.2));
#26735=CARTESIAN_POINT('Ctrl Pts',(0.0585811257615177,0.0985345138164694,
-0.199514986736451));
#26736=CARTESIAN_POINT('Ctrl Pts',(0.0577350269189626,0.1,-0.199));
#26737=CARTESIAN_POINT('',(0.0543747087933691,0.1,-0.2));
#26738=CARTESIAN_POINT('Origin',(0.,0.,-0.2));
#26739=CARTESIAN_POINT('Ctrl Pts',(0.0577350269189626,0.1,-0.199));
#26740=CARTESIAN_POINT('Ctrl Pts',(0.0560428292338471,0.1,-0.199514986736452));
#26741=CARTESIAN_POINT('Ctrl Pts',(0.0543747087933691,0.1,-0.2));
#26742=CARTESIAN_POINT('',(-0.0543747087933691,0.1,-0.2));
#26743=CARTESIAN_POINT('Ctrl Pts',(-0.0543747087933691,0.1,-0.2));
#26744=CARTESIAN_POINT('Ctrl Pts',(-0.0560428292338464,0.1,-0.199514986736453));
#26745=CARTESIAN_POINT('Ctrl Pts',(-0.0577350269189626,0.1,-0.199));
#26746=CARTESIAN_POINT('',(-0.0594151859817593,0.0970898791384387,-0.2));
#26747=CARTESIAN_POINT('Origin',(0.,0.,-0.2));
#26748=CARTESIAN_POINT('Ctrl Pts',(-0.0577350269189626,0.1,-0.199));
#26749=CARTESIAN_POINT('Ctrl Pts',(-0.0585811257615179,0.0985345138164689,
-0.199514986736451));
#26750=CARTESIAN_POINT('Ctrl Pts',(-0.0594151859817593,0.0970898791384388,
-0.2));
#26751=CARTESIAN_POINT('',(-0.113789894775128,0.0029101208615613,-0.2));
#26752=CARTESIAN_POINT('Ctrl Pts',(-0.113789894775128,0.00291012086156131,
-0.2));
#26753=CARTESIAN_POINT('Ctrl Pts',(-0.11462395499537,0.00146548618353128,
-0.199514986736451));
#26754=CARTESIAN_POINT('Ctrl Pts',(-0.115470053837925,2.08166817117217E-17,
-0.199));
#26755=CARTESIAN_POINT('Origin',(0.,0.,-0.2));
#26756=CARTESIAN_POINT('Origin',(-0.115470053837925,1.38777878078145E-17,
0.));
#26757=CARTESIAN_POINT('',(-0.0577350269189626,0.1,0.));
#26758=CARTESIAN_POINT('',(-0.0577350269189626,0.1,0.));
#26759=CARTESIAN_POINT('',(-0.115470053837925,1.41410031829988E-17,0.));
#26760=CARTESIAN_POINT('',(-0.101036297108185,0.025,0.));
#26761=CARTESIAN_POINT('',(-0.115470053837925,1.41410031829988E-17,0.));
#26762=CARTESIAN_POINT('Origin',(-0.115470053837925,1.38777878078145E-17,
0.));
#26763=CARTESIAN_POINT('',(-0.115470053837925,1.38777878078145E-17,-0.2));
#26764=CARTESIAN_POINT('',(-0.115470053837925,1.41410031829988E-17,0.));
#26765=CARTESIAN_POINT('',(-0.0577350269189626,0.1,-0.2));
#26766=CARTESIAN_POINT('Origin',(-0.0577350269189626,0.1,0.));
#26767=CARTESIAN_POINT('',(0.0577350269189626,0.1,0.));
#26768=CARTESIAN_POINT('',(0.0577350269189626,0.1,0.));
#26769=CARTESIAN_POINT('',(-0.0288675134594813,0.1,0.));
#26770=CARTESIAN_POINT('Origin',(-0.0577350269189626,0.1,0.));
#26771=CARTESIAN_POINT('',(0.0577350269189626,0.1,-0.2));
#26772=CARTESIAN_POINT('',(0.0577350269189626,0.1,-0.2));
#26773=CARTESIAN_POINT('',(0.0577350269189626,0.1,0.));
#26774=CARTESIAN_POINT('Origin',(-0.0577350269189626,0.1,0.));
#26775=CARTESIAN_POINT('',(-0.0577350269189626,0.1,-0.2));
#26776=CARTESIAN_POINT('',(-0.0577350269189626,0.1,0.));
#26777=CARTESIAN_POINT('',(0.0577350269189626,0.1,-0.2));
#26778=CARTESIAN_POINT('Origin',(-0.0577350269189626,-0.1,0.));
#26779=CARTESIAN_POINT('',(-0.0577350269189626,-0.1,0.));
#26780=CARTESIAN_POINT('',(-0.0721687836487033,-0.075,0.));
#26781=CARTESIAN_POINT('',(-0.0577350269189626,-0.1,0.));
#26782=CARTESIAN_POINT('Origin',(-0.0577350269189626,-0.1,0.));
#26783=CARTESIAN_POINT('',(-0.0577350269189626,-0.1,-0.2));
#26784=CARTESIAN_POINT('',(-0.0577350269189626,-0.1,0.));
#26785=CARTESIAN_POINT('',(-0.115470053837925,1.41410031829988E-17,-0.2));
#26786=CARTESIAN_POINT('Origin',(0.0577350269189626,0.1,0.));
#26787=CARTESIAN_POINT('',(0.115470053837925,0.,0.));
#26788=CARTESIAN_POINT('',(0.115470053837925,0.,0.));
#26789=CARTESIAN_POINT('',(0.0721687836487032,0.075,0.));
#26790=CARTESIAN_POINT('Origin',(0.0577350269189626,0.1,0.));
#26791=CARTESIAN_POINT('',(0.115470053837925,0.,-0.2));
#26792=CARTESIAN_POINT('',(0.115470053837925,0.,-0.2));
#26793=CARTESIAN_POINT('',(0.115470053837925,0.,0.));
#26794=CARTESIAN_POINT('Origin',(0.0577350269189626,0.1,0.));
#26795=CARTESIAN_POINT('',(0.115470053837925,0.,-0.2));
#26796=CARTESIAN_POINT('Origin',(0.,0.,-0.2));
#26797=CARTESIAN_POINT('',(-0.0577350269189626,0.1,-0.2));
#26798=CARTESIAN_POINT('Origin',(0.,0.,-0.2));
#26799=CARTESIAN_POINT('Origin',(0.,0.,-0.2));
#26800=CARTESIAN_POINT('',(0.0577350269189626,-0.1,-0.2));
#26801=CARTESIAN_POINT('Origin',(0.,0.,-0.2));
#26802=CARTESIAN_POINT('',(0.0577350269189626,-0.1,-0.2));
#26803=CARTESIAN_POINT('',(-0.0577350269189626,-0.1,-0.2));
#26804=CARTESIAN_POINT('',(0.0577350269189626,-0.1,-0.2));
#26805=CARTESIAN_POINT('Origin',(0.,0.,-0.2));
#26806=CARTESIAN_POINT('',(-0.0577350269189626,-0.1,-0.2));
#26807=CARTESIAN_POINT('Origin',(0.,0.,-0.2));
#26808=CARTESIAN_POINT('',(-0.115470053837925,1.41410031829988E-17,-0.2));
#26809=CARTESIAN_POINT('Origin',(0.115470053837925,0.,0.));
#26810=CARTESIAN_POINT('',(0.0577350269189626,-0.1,0.));
#26811=CARTESIAN_POINT('',(0.0577350269189626,-0.1,0.));
#26812=CARTESIAN_POINT('',(0.101036297108185,-0.025,0.));
#26813=CARTESIAN_POINT('Origin',(0.115470053837925,0.,0.));
#26814=CARTESIAN_POINT('',(0.0577350269189626,-0.1,0.));
#26815=CARTESIAN_POINT('Origin',(0.115470053837925,0.,0.));
#26816=CARTESIAN_POINT('Origin',(0.0577350269189626,-0.1,0.));
#26817=CARTESIAN_POINT('Origin',(0.0577350269189626,-0.1,0.));
#26818=CARTESIAN_POINT('',(0.0288675134594813,-0.1,0.));
#26819=CARTESIAN_POINT('Origin',(-0.115470053837925,1.38777878078145E-17,
0.));
#26820=CARTESIAN_POINT('Origin',(-0.0577350269189626,-0.1,0.));
#26821=CARTESIAN_POINT('Origin',(0.0577350269189626,-0.1,0.));
#26822=CARTESIAN_POINT('Origin',(0.125,0.,-0.4));
#26823=CARTESIAN_POINT('',(-0.125,-1.53080849893419E-17,-0.4));
#26824=CARTESIAN_POINT('Origin',(0.,0.,-0.4));
#26825=CARTESIAN_POINT('Origin',(0.,0.,-0.375));
#26826=CARTESIAN_POINT('',(-0.1625,-1.99005104861445E-17,-0.375));
#26827=CARTESIAN_POINT('Origin',(0.,0.,-0.19));
#26828=CARTESIAN_POINT('Origin',(0.,0.,-0.0254));
#26829=CARTESIAN_POINT('Origin',(0.,0.,-0.015));
#26830=CARTESIAN_POINT('',(-0.17,-2.0818995585505E-17,-1.73472347597681E-18));
#26831=CARTESIAN_POINT('Origin',(0.,0.,0.));
#26832=CARTESIAN_POINT('',(-0.185,-2.2655965784226E-17,-0.015));
#26833=CARTESIAN_POINT('Origin',(0.,0.,0.));
#38588=UNCERTAINTY_MEASURE_WITH_UNIT(LENGTH_MEASURE(0.001),#38612,
'DISTANCE_ACCURACY_VALUE',
'Maximum model space distance between geometric entities at asserted c
onnectivities');
#38595=UNCERTAINTY_MEASURE_WITH_UNIT(LENGTH_MEASURE(0.001),#38612,
'DISTANCE_ACCURACY_VALUE',
'Maximum model space distance between geometric entities at asserted c
onnectivities');
#38604=(
GEOMETRIC_REPRESENTATION_CONTEXT(3)
GLOBAL_UNCERTAINTY_ASSIGNED_CONTEXT((#38588))
GLOBAL_UNIT_ASSIGNED_CONTEXT((#38612,#38614,#38615))
REPRESENTATION_CONTEXT('','3D')
);
#38611=(
GEOMETRIC_REPRESENTATION_CONTEXT(3)
GLOBAL_UNCERTAINTY_ASSIGNED_CONTEXT((#38595))
GLOBAL_UNIT_ASSIGNED_CONTEXT((#38612,#38614,#38615))
REPRESENTATION_CONTEXT('','3D')
);
#38612=(
LENGTH_UNIT()
NAMED_UNIT(*)
SI_UNIT(.CENTI.,.METRE.)
);
#38614=(
NAMED_UNIT(*)
PLANE_ANGLE_UNIT()
SI_UNIT($,.RADIAN.)
);
#38615=(
NAMED_UNIT(*)
SI_UNIT($,.STERADIAN.)
SOLID_ANGLE_UNIT()
);
#38624=SHAPE_DEFINITION_REPRESENTATION(#38639,#38675);
#38639=PRODUCT_DEFINITION_SHAPE('',$,#38691);
#38675=SHAPE_REPRESENTATION('',(#16909),#38604);
#38682=PRODUCT_DEFINITION_CONTEXT('part definition',#38729,'design');
#38691=PRODUCT_DEFINITION('2026-10-19-02-32-13-450',
'14_ISO_4026_M4x4_Set_Screw',#38706,#38682);
#38706=PRODUCT_DEFINITION_FORMATION('',$,#38739);
#38729=APPLICATION_CONTEXT(
'Core Data for Automotive Mechanical Design Process');
#38730=PRODUCT_CONTEXT('part definition',#38729,'mechanical');
#38739=PRODUCT('2026-10-19-02-32-13-450','14_ISO_4026_M4x4_Set_Screw',$,
(#38730));
#38879=COLOUR_RGB('Black',0.12,0.14,0.17);
#38880=FILL_AREA_STYLE_COLOUR('',#38879);
#38881=FILL_AREA_STYLE('',(#38880));
#38882=SURFACE_STYLE_FILL_AREA(#38881);
#38883=SURFACE_SIDE_STYLE('',(#38882));
#38884=SURFACE_STYLE_USAGE(.BOTH.,#38883);
#38885=PRESENTATION_STYLE_ASSIGNMENT((#38884));
ENDSEC;
END-ISO-10303-21;
